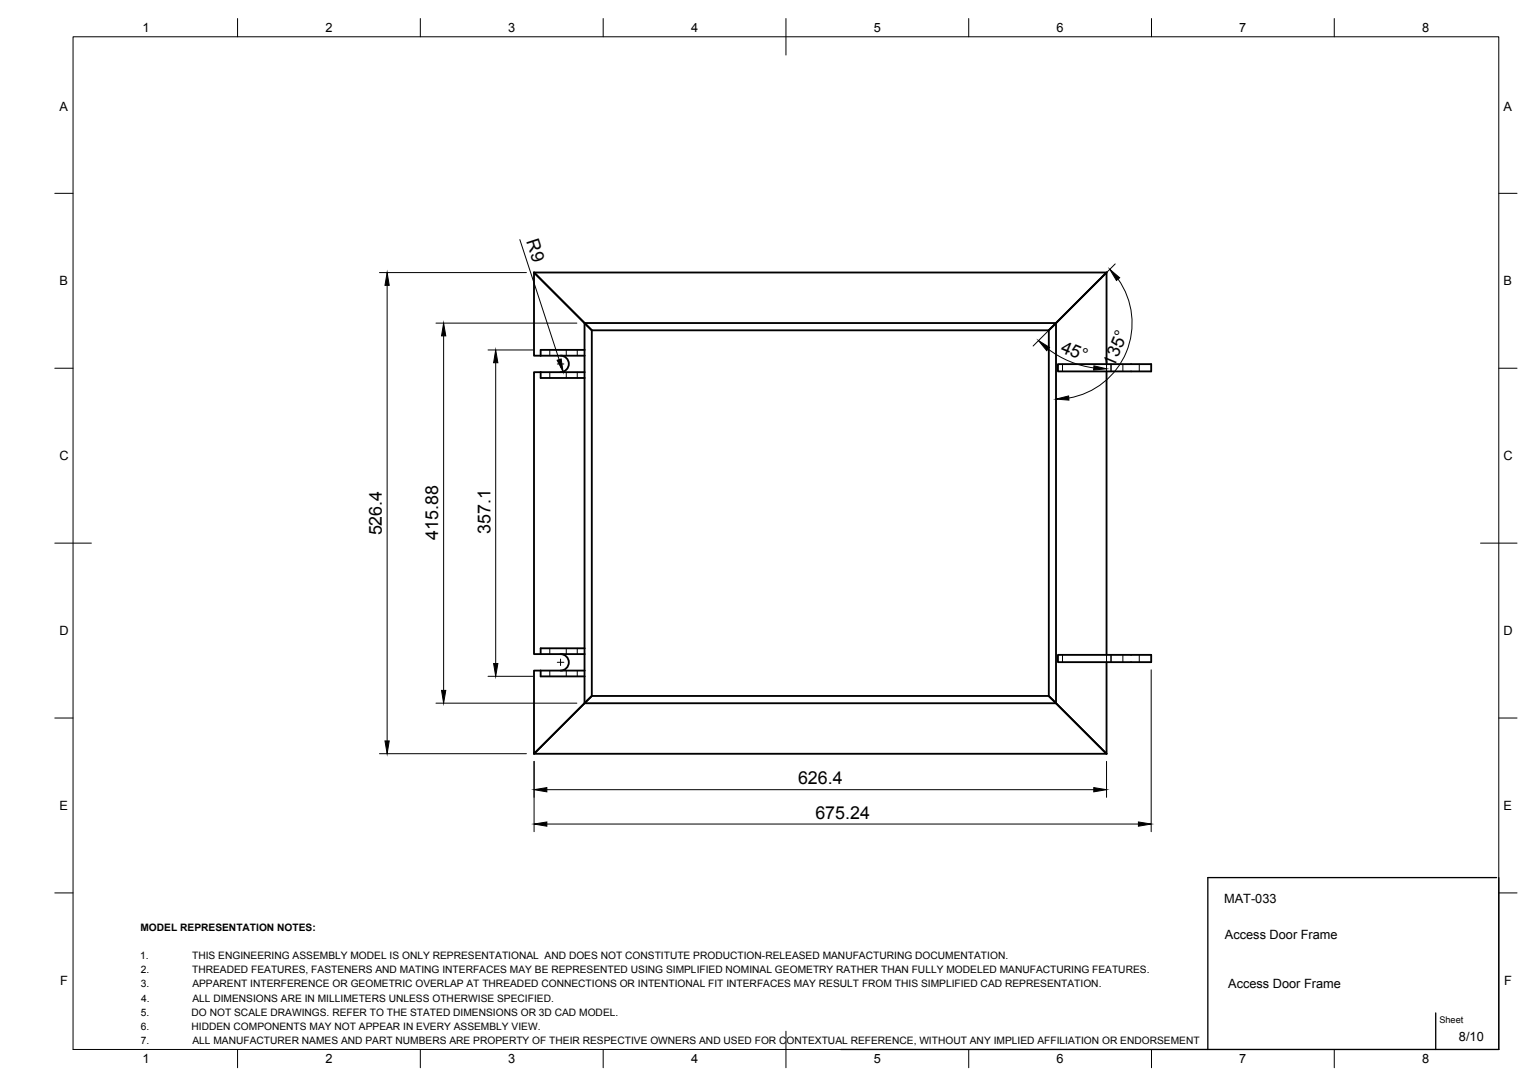
ISO-10303-21;
HEADER;
/* Generated by software containing ST-Developer
 * from STEP Tools, Inc. (www.steptools.com) 
 */

FILE_DESCRIPTION(
/* description */ ('STEP AP214'),
/* implementation_level */ '2;1');

FILE_NAME(
/* name */ 'Access Door Frame.step',
/* time_stamp */ '2026-11-14T07:13:32-08:00',
/* author */ (''),
/* organization */ (''),
/* preprocessor_version */ 'ST-DEVELOPER v20.2',
/* originating_system */ 'Autodesk Translation Framework v15.17.0.0',
/* authorisation */ '');

FILE_SCHEMA (('AUTOMOTIVE_DESIGN { 1 0 10303 214 3 1 1 }'));
ENDSEC;

DATA;
#10=MECHANICAL_DESIGN_GEOMETRIC_PRESENTATION_REPRESENTATION('',(#1305,#1306,#1307,#1308,#1309,#1310,#1311,#1312,#1313,#1314),#32903);
#644=ELLIPSE('',#16043,10.9424774388658,7.73750000000281);
#645=ELLIPSE('',#16044,11.2253201513379,7.93750000000103);
#646=ELLIPSE('',#16045,10.9424774388637,7.73750000000177);
#647=ELLIPSE('',#16047,10.9424774388587,7.73749999999781);
#648=ELLIPSE('',#16048,11.2253201513381,7.93750000000136);
#649=ELLIPSE('',#16049,10.9424774388615,7.73749999999964);
#650=ELLIPSE('',#16060,10.9424774388615,7.73749999999999);
#651=ELLIPSE('',#16061,11.2253201513371,7.93750000000052);
#652=ELLIPSE('',#16062,10.9424774388621,7.73750000000035);
#653=ELLIPSE('',#16064,10.9424774388604,7.73749999999896);
#654=ELLIPSE('',#16065,11.2253201513326,7.93749999999674);
#655=ELLIPSE('',#16066,10.9424774388621,7.73750000000041);
#656=ELLIPSE('',#16077,10.9424774388579,7.73749999999704);
#657=ELLIPSE('',#16078,11.2253201513353,7.9374999999993);
#658=ELLIPSE('',#16079,10.9424774388611,7.73749999999964);
#659=ELLIPSE('',#16081,10.9424774388619,7.73750000000076);
#660=ELLIPSE('',#16082,11.2253201513349,7.93749999999867);
#661=ELLIPSE('',#16083,10.942477438863,7.73750000000083);
#662=ELLIPSE('',#16160,10.9424774388598,7.7374999999982);
#663=ELLIPSE('',#16164,10.9424774388633,7.73750000000104);
#664=ELLIPSE('',#16165,11.225320151339,7.9375000000018);
#665=ELLIPSE('',#16166,10.9424774388576,7.73749999999669);
#666=ELLIPSE('',#16168,10.9424774388584,7.73749999999717);
#667=ELLIPSE('',#16169,11.2253201513371,7.93750000000039);
#674=SHAPE_REPRESENTATION_RELATIONSHIP('SRR','None',#33016,#688);
#688=ADVANCED_BREP_SHAPE_REPRESENTATION('',(#1394,#1395,#1396,#1397,#1398,
#1399,#1400,#1401,#1402,#1403),#32891);
#820=CIRCLE('',#16094,9.00000000000001);
#821=CIRCLE('',#16095,9.00000000000001);
#822=CIRCLE('',#16097,22.);
#823=CIRCLE('',#16098,22.);
#824=CIRCLE('',#16100,5.);
#825=CIRCLE('',#16101,5.);
#826=CIRCLE('',#16109,9.00000000000001);
#827=CIRCLE('',#16110,9.00000000000001);
#828=CIRCLE('',#16112,19.);
#829=CIRCLE('',#16114,19.);
#830=CIRCLE('',#16122,9.00000000000001);
#831=CIRCLE('',#16123,9.00000000000001);
#832=CIRCLE('',#16125,22.);
#833=CIRCLE('',#16126,22.);
#834=CIRCLE('',#16128,5.);
#835=CIRCLE('',#16129,5.);
#836=CIRCLE('',#16137,9.00000000000001);
#837=CIRCLE('',#16138,9.00000000000001);
#838=CIRCLE('',#16140,19.);
#839=CIRCLE('',#16142,19.);
#840=CIRCLE('',#16150,9.00000000000001);
#841=CIRCLE('',#16151,9.00000000000001);
#842=CIRCLE('',#16153,9.00000000000006);
#843=CIRCLE('',#16154,9.00000000000001);
#844=CIRCLE('',#16156,7.73750000000001);
#845=CIRCLE('',#16157,7.73750000000001);
#846=CIRCLE('',#16159,7.73750000000001);
#847=CIRCLE('',#16178,7.73750000000001);
#848=CIRCLE('',#16185,9.00000000000001);
#849=CIRCLE('',#16186,9.00000000000001);
#850=CIRCLE('',#16188,19.);
#851=CIRCLE('',#16190,19.);
#852=CIRCLE('',#16198,9.00000000000001);
#853=CIRCLE('',#16199,9.00000000000001);
#854=CIRCLE('',#16201,19.);
#855=CIRCLE('',#16203,19.);
#1141=CYLINDRICAL_SURFACE('',#16053,7.73749999999998);
#1142=CYLINDRICAL_SURFACE('',#16055,7.93749999999999);
#1143=CYLINDRICAL_SURFACE('',#16057,7.73750000000001);
#1144=CYLINDRICAL_SURFACE('',#16070,7.73749999999998);
#1145=CYLINDRICAL_SURFACE('',#16072,7.93750000000002);
#1146=CYLINDRICAL_SURFACE('',#16074,7.73750000000001);
#1147=CYLINDRICAL_SURFACE('',#16087,7.73749999999998);
#1148=CYLINDRICAL_SURFACE('',#16089,7.93750000000002);
#1149=CYLINDRICAL_SURFACE('',#16091,7.73750000000001);
#1150=CYLINDRICAL_SURFACE('',#16093,9.00000000000001);
#1151=CYLINDRICAL_SURFACE('',#16096,22.);
#1152=CYLINDRICAL_SURFACE('',#16099,5.);
#1153=CYLINDRICAL_SURFACE('',#16108,9.00000000000001);
#1154=CYLINDRICAL_SURFACE('',#16118,19.);
#1155=CYLINDRICAL_SURFACE('',#16121,9.00000000000001);
#1156=CYLINDRICAL_SURFACE('',#16124,22.);
#1157=CYLINDRICAL_SURFACE('',#16127,5.);
#1158=CYLINDRICAL_SURFACE('',#16136,9.00000000000001);
#1159=CYLINDRICAL_SURFACE('',#16146,19.);
#1160=CYLINDRICAL_SURFACE('',#16149,9.00000000000001);
#1161=CYLINDRICAL_SURFACE('',#16152,9.00000000000006);
#1162=CYLINDRICAL_SURFACE('',#16155,7.73750000000001);
#1163=CYLINDRICAL_SURFACE('',#16158,7.73750000000001);
#1164=CYLINDRICAL_SURFACE('',#16173,7.73749999999998);
#1165=CYLINDRICAL_SURFACE('',#16175,7.93749999999999);
#1166=CYLINDRICAL_SURFACE('',#16177,7.73750000000001);
#1167=CYLINDRICAL_SURFACE('',#16184,9.00000000000001);
#1168=CYLINDRICAL_SURFACE('',#16194,19.);
#1169=CYLINDRICAL_SURFACE('',#16197,9.00000000000001);
#1170=CYLINDRICAL_SURFACE('',#16207,19.);
#1305=STYLED_ITEM('',(#33098),#1394);
#1306=STYLED_ITEM('',(#33098),#1395);
#1307=STYLED_ITEM('',(#33098),#1396);
#1308=STYLED_ITEM('',(#33098),#1397);
#1309=STYLED_ITEM('',(#33098),#1398);
#1310=STYLED_ITEM('',(#33098),#1399);
#1311=STYLED_ITEM('',(#33098),#1400);
#1312=STYLED_ITEM('',(#33098),#1401);
#1313=STYLED_ITEM('',(#33098),#1402);
#1314=STYLED_ITEM('',(#33098),#1403);
#1394=MANIFOLD_SOLID_BREP('Body1',#15553);
#1395=MANIFOLD_SOLID_BREP('Body2',#15554);
#1396=MANIFOLD_SOLID_BREP('Body3',#15555);
#1397=MANIFOLD_SOLID_BREP('Body4',#15556);
#1398=MANIFOLD_SOLID_BREP('Body5',#15557);
#1399=MANIFOLD_SOLID_BREP('Body6',#15558);
#1400=MANIFOLD_SOLID_BREP('Body7',#15559);
#1401=MANIFOLD_SOLID_BREP('Body8',#15560);
#1402=MANIFOLD_SOLID_BREP('Body9',#15561);
#1403=MANIFOLD_SOLID_BREP('Body10',#15562);
#1579=FACE_BOUND('',#2856,.T.);
#1580=FACE_BOUND('',#2858,.T.);
#1581=FACE_BOUND('',#2861,.T.);
#1582=FACE_BOUND('',#2863,.T.);
#1583=FACE_BOUND('',#2878,.T.);
#1584=FACE_BOUND('',#2880,.T.);
#1585=FACE_BOUND('',#2883,.T.);
#1586=FACE_BOUND('',#2885,.T.);
#1587=FACE_BOUND('',#2915,.T.);
#1588=FACE_BOUND('',#2917,.T.);
#1589=FACE_BOUND('',#2926,.T.);
#1590=FACE_BOUND('',#2928,.T.);
#1810=FACE_OUTER_BOUND('',#2815,.T.);
#1811=FACE_OUTER_BOUND('',#2816,.T.);
#1812=FACE_OUTER_BOUND('',#2817,.T.);
#1813=FACE_OUTER_BOUND('',#2818,.T.);
#1814=FACE_OUTER_BOUND('',#2819,.T.);
#1815=FACE_OUTER_BOUND('',#2820,.T.);
#1816=FACE_OUTER_BOUND('',#2821,.T.);
#1817=FACE_OUTER_BOUND('',#2822,.T.);
#1818=FACE_OUTER_BOUND('',#2823,.T.);
#1819=FACE_OUTER_BOUND('',#2824,.T.);
#1820=FACE_OUTER_BOUND('',#2825,.T.);
#1821=FACE_OUTER_BOUND('',#2826,.T.);
#1822=FACE_OUTER_BOUND('',#2827,.T.);
#1823=FACE_OUTER_BOUND('',#2828,.T.);
#1824=FACE_OUTER_BOUND('',#2829,.T.);
#1825=FACE_OUTER_BOUND('',#2830,.T.);
#1826=FACE_OUTER_BOUND('',#2831,.T.);
#1827=FACE_OUTER_BOUND('',#2832,.T.);
#1828=FACE_OUTER_BOUND('',#2833,.T.);
#1829=FACE_OUTER_BOUND('',#2834,.T.);
#1830=FACE_OUTER_BOUND('',#2835,.T.);
#1831=FACE_OUTER_BOUND('',#2836,.T.);
#1832=FACE_OUTER_BOUND('',#2837,.T.);
#1833=FACE_OUTER_BOUND('',#2838,.T.);
#1834=FACE_OUTER_BOUND('',#2839,.T.);
#1835=FACE_OUTER_BOUND('',#2840,.T.);
#1836=FACE_OUTER_BOUND('',#2841,.T.);
#1837=FACE_OUTER_BOUND('',#2842,.T.);
#1838=FACE_OUTER_BOUND('',#2843,.T.);
#1839=FACE_OUTER_BOUND('',#2844,.T.);
#1840=FACE_OUTER_BOUND('',#2845,.T.);
#1841=FACE_OUTER_BOUND('',#2846,.T.);
#1842=FACE_OUTER_BOUND('',#2847,.T.);
#1843=FACE_OUTER_BOUND('',#2848,.T.);
#1844=FACE_OUTER_BOUND('',#2849,.T.);
#1845=FACE_OUTER_BOUND('',#2850,.T.);
#1846=FACE_OUTER_BOUND('',#2851,.T.);
#1847=FACE_OUTER_BOUND('',#2852,.T.);
#1848=FACE_OUTER_BOUND('',#2853,.T.);
#1849=FACE_OUTER_BOUND('',#2854,.T.);
#1850=FACE_OUTER_BOUND('',#2855,.T.);
#1851=FACE_OUTER_BOUND('',#2857,.T.);
#1852=FACE_OUTER_BOUND('',#2859,.T.);
#1853=FACE_OUTER_BOUND('',#2860,.T.);
#1854=FACE_OUTER_BOUND('',#2862,.T.);
#1855=FACE_OUTER_BOUND('',#2864,.T.);
#1856=FACE_OUTER_BOUND('',#2865,.T.);
#1857=FACE_OUTER_BOUND('',#2866,.T.);
#1858=FACE_OUTER_BOUND('',#2867,.T.);
#1859=FACE_OUTER_BOUND('',#2868,.T.);
#1860=FACE_OUTER_BOUND('',#2869,.T.);
#1861=FACE_OUTER_BOUND('',#2870,.T.);
#1862=FACE_OUTER_BOUND('',#2871,.T.);
#1863=FACE_OUTER_BOUND('',#2872,.T.);
#1864=FACE_OUTER_BOUND('',#2873,.T.);
#1865=FACE_OUTER_BOUND('',#2874,.T.);
#1866=FACE_OUTER_BOUND('',#2875,.T.);
#1867=FACE_OUTER_BOUND('',#2876,.T.);
#1868=FACE_OUTER_BOUND('',#2877,.T.);
#1869=FACE_OUTER_BOUND('',#2879,.T.);
#1870=FACE_OUTER_BOUND('',#2881,.T.);
#1871=FACE_OUTER_BOUND('',#2882,.T.);
#1872=FACE_OUTER_BOUND('',#2884,.T.);
#1873=FACE_OUTER_BOUND('',#2886,.T.);
#1874=FACE_OUTER_BOUND('',#2887,.T.);
#1875=FACE_OUTER_BOUND('',#2888,.T.);
#1876=FACE_OUTER_BOUND('',#2889,.T.);
#1877=FACE_OUTER_BOUND('',#2890,.T.);
#1878=FACE_OUTER_BOUND('',#2891,.T.);
#1879=FACE_OUTER_BOUND('',#2892,.T.);
#1880=FACE_OUTER_BOUND('',#2893,.T.);
#1881=FACE_OUTER_BOUND('',#2894,.T.);
#1882=FACE_OUTER_BOUND('',#2895,.T.);
#1883=FACE_OUTER_BOUND('',#2896,.T.);
#1884=FACE_OUTER_BOUND('',#2897,.T.);
#1885=FACE_OUTER_BOUND('',#2898,.T.);
#1886=FACE_OUTER_BOUND('',#2899,.T.);
#1887=FACE_OUTER_BOUND('',#2900,.T.);
#1888=FACE_OUTER_BOUND('',#2901,.T.);
#1889=FACE_OUTER_BOUND('',#2902,.T.);
#1890=FACE_OUTER_BOUND('',#2903,.T.);
#1891=FACE_OUTER_BOUND('',#2904,.T.);
#1892=FACE_OUTER_BOUND('',#2905,.T.);
#1893=FACE_OUTER_BOUND('',#2906,.T.);
#1894=FACE_OUTER_BOUND('',#2907,.T.);
#1895=FACE_OUTER_BOUND('',#2908,.T.);
#1896=FACE_OUTER_BOUND('',#2909,.T.);
#1897=FACE_OUTER_BOUND('',#2910,.T.);
#1898=FACE_OUTER_BOUND('',#2911,.T.);
#1899=FACE_OUTER_BOUND('',#2912,.T.);
#1900=FACE_OUTER_BOUND('',#2913,.T.);
#1901=FACE_OUTER_BOUND('',#2914,.T.);
#1902=FACE_OUTER_BOUND('',#2916,.T.);
#1903=FACE_OUTER_BOUND('',#2918,.T.);
#1904=FACE_OUTER_BOUND('',#2919,.T.);
#1905=FACE_OUTER_BOUND('',#2920,.T.);
#1906=FACE_OUTER_BOUND('',#2921,.T.);
#1907=FACE_OUTER_BOUND('',#2922,.T.);
#1908=FACE_OUTER_BOUND('',#2923,.T.);
#1909=FACE_OUTER_BOUND('',#2924,.T.);
#1910=FACE_OUTER_BOUND('',#2925,.T.);
#1911=FACE_OUTER_BOUND('',#2927,.T.);
#1912=FACE_OUTER_BOUND('',#2929,.T.);
#1913=FACE_OUTER_BOUND('',#2930,.T.);
#1914=FACE_OUTER_BOUND('',#2931,.T.);
#1915=FACE_OUTER_BOUND('',#2932,.T.);
#1916=FACE_OUTER_BOUND('',#2933,.T.);
#1917=FACE_OUTER_BOUND('',#2934,.T.);
#2815=EDGE_LOOP('',(#10543,#10544,#10545,#10546,#10547,#10548,#10549,#10550,
#10551));
#2816=EDGE_LOOP('',(#10552,#10553,#10554,#10555,#10556,#10557,#10558,#10559,
#10560));
#2817=EDGE_LOOP('',(#10561,#10562,#10563,#10564));
#2818=EDGE_LOOP('',(#10565,#10566,#10567,#10568));
#2819=EDGE_LOOP('',(#10569,#10570,#10571,#10572));
#2820=EDGE_LOOP('',(#10573,#10574,#10575,#10576));
#2821=EDGE_LOOP('',(#10577,#10578,#10579,#10580));
#2822=EDGE_LOOP('',(#10581,#10582,#10583,#10584));
#2823=EDGE_LOOP('',(#10585,#10586,#10587,#10588));
#2824=EDGE_LOOP('',(#10589,#10590,#10591,#10592));
#2825=EDGE_LOOP('',(#10593,#10594,#10595,#10596));
#2826=EDGE_LOOP('',(#10597,#10598,#10599,#10600,#10601,#10602,#10603,#10604,
#10605));
#2827=EDGE_LOOP('',(#10606,#10607,#10608,#10609,#10610,#10611,#10612,#10613,
#10614));
#2828=EDGE_LOOP('',(#10615,#10616,#10617,#10618));
#2829=EDGE_LOOP('',(#10619,#10620,#10621,#10622));
#2830=EDGE_LOOP('',(#10623,#10624,#10625,#10626));
#2831=EDGE_LOOP('',(#10627,#10628,#10629,#10630));
#2832=EDGE_LOOP('',(#10631,#10632,#10633,#10634));
#2833=EDGE_LOOP('',(#10635,#10636,#10637,#10638));
#2834=EDGE_LOOP('',(#10639,#10640,#10641,#10642));
#2835=EDGE_LOOP('',(#10643,#10644,#10645,#10646));
#2836=EDGE_LOOP('',(#10647,#10648,#10649,#10650));
#2837=EDGE_LOOP('',(#10651,#10652,#10653,#10654,#10655,#10656,#10657,#10658,
#10659));
#2838=EDGE_LOOP('',(#10660,#10661,#10662,#10663,#10664,#10665,#10666,#10667,
#10668));
#2839=EDGE_LOOP('',(#10669,#10670,#10671,#10672));
#2840=EDGE_LOOP('',(#10673,#10674,#10675,#10676));
#2841=EDGE_LOOP('',(#10677,#10678,#10679,#10680));
#2842=EDGE_LOOP('',(#10681,#10682,#10683,#10684));
#2843=EDGE_LOOP('',(#10685,#10686,#10687,#10688));
#2844=EDGE_LOOP('',(#10689,#10690,#10691,#10692));
#2845=EDGE_LOOP('',(#10693,#10694,#10695,#10696));
#2846=EDGE_LOOP('',(#10697,#10698,#10699,#10700));
#2847=EDGE_LOOP('',(#10701,#10702,#10703,#10704));
#2848=EDGE_LOOP('',(#10705,#10706,#10707,#10708));
#2849=EDGE_LOOP('',(#10709,#10710,#10711,#10712));
#2850=EDGE_LOOP('',(#10713,#10714,#10715,#10716));
#2851=EDGE_LOOP('',(#10717,#10718,#10719,#10720));
#2852=EDGE_LOOP('',(#10721,#10722,#10723,#10724));
#2853=EDGE_LOOP('',(#10725,#10726,#10727,#10728));
#2854=EDGE_LOOP('',(#10729,#10730,#10731,#10732));
#2855=EDGE_LOOP('',(#10733,#10734,#10735,#10736,#10737,#10738));
#2856=EDGE_LOOP('',(#10739));
#2857=EDGE_LOOP('',(#10740,#10741,#10742,#10743,#10744,#10745));
#2858=EDGE_LOOP('',(#10746));
#2859=EDGE_LOOP('',(#10747,#10748,#10749,#10750));
#2860=EDGE_LOOP('',(#10751,#10752,#10753,#10754,#10755,#10756));
#2861=EDGE_LOOP('',(#10757));
#2862=EDGE_LOOP('',(#10758,#10759,#10760,#10761,#10762,#10763));
#2863=EDGE_LOOP('',(#10764));
#2864=EDGE_LOOP('',(#10765,#10766,#10767,#10768));
#2865=EDGE_LOOP('',(#10769,#10770,#10771,#10772));
#2866=EDGE_LOOP('',(#10773,#10774,#10775,#10776));
#2867=EDGE_LOOP('',(#10777,#10778,#10779,#10780));
#2868=EDGE_LOOP('',(#10781,#10782,#10783,#10784));
#2869=EDGE_LOOP('',(#10785,#10786,#10787,#10788));
#2870=EDGE_LOOP('',(#10789,#10790,#10791,#10792));
#2871=EDGE_LOOP('',(#10793,#10794,#10795,#10796));
#2872=EDGE_LOOP('',(#10797,#10798,#10799,#10800));
#2873=EDGE_LOOP('',(#10801,#10802,#10803,#10804));
#2874=EDGE_LOOP('',(#10805,#10806,#10807,#10808));
#2875=EDGE_LOOP('',(#10809,#10810,#10811,#10812));
#2876=EDGE_LOOP('',(#10813,#10814,#10815,#10816));
#2877=EDGE_LOOP('',(#10817,#10818,#10819,#10820,#10821,#10822));
#2878=EDGE_LOOP('',(#10823));
#2879=EDGE_LOOP('',(#10824,#10825,#10826,#10827,#10828,#10829));
#2880=EDGE_LOOP('',(#10830));
#2881=EDGE_LOOP('',(#10831,#10832,#10833,#10834));
#2882=EDGE_LOOP('',(#10835,#10836,#10837,#10838,#10839,#10840));
#2883=EDGE_LOOP('',(#10841));
#2884=EDGE_LOOP('',(#10842,#10843,#10844,#10845,#10846,#10847));
#2885=EDGE_LOOP('',(#10848));
#2886=EDGE_LOOP('',(#10849,#10850,#10851,#10852));
#2887=EDGE_LOOP('',(#10853,#10854,#10855,#10856));
#2888=EDGE_LOOP('',(#10857,#10858,#10859,#10860));
#2889=EDGE_LOOP('',(#10861,#10862,#10863,#10864));
#2890=EDGE_LOOP('',(#10865,#10866,#10867,#10868));
#2891=EDGE_LOOP('',(#10869,#10870,#10871,#10872));
#2892=EDGE_LOOP('',(#10873,#10874,#10875,#10876));
#2893=EDGE_LOOP('',(#10877,#10878,#10879,#10880));
#2894=EDGE_LOOP('',(#10881,#10882,#10883,#10884));
#2895=EDGE_LOOP('',(#10885,#10886,#10887,#10888));
#2896=EDGE_LOOP('',(#10889,#10890,#10891,#10892));
#2897=EDGE_LOOP('',(#10893,#10894,#10895,#10896));
#2898=EDGE_LOOP('',(#10897,#10898,#10899,#10900,#10901,#10902,#10903,#10904,
#10905));
#2899=EDGE_LOOP('',(#10906,#10907,#10908,#10909,#10910,#10911,#10912,#10913,
#10914));
#2900=EDGE_LOOP('',(#10915,#10916,#10917,#10918,#10919,#10920,#10921,#10922,
#10923,#10924,#10925,#10926));
#2901=EDGE_LOOP('',(#10927,#10928,#10929,#10930));
#2902=EDGE_LOOP('',(#10931,#10932,#10933,#10934));
#2903=EDGE_LOOP('',(#10935,#10936,#10937,#10938));
#2904=EDGE_LOOP('',(#10939,#10940,#10941,#10942));
#2905=EDGE_LOOP('',(#10943,#10944,#10945,#10946));
#2906=EDGE_LOOP('',(#10947,#10948,#10949,#10950,#10951,#10952,#10953,#10954,
#10955,#10956,#10957,#10958));
#2907=EDGE_LOOP('',(#10959,#10960,#10961,#10962));
#2908=EDGE_LOOP('',(#10963,#10964,#10965,#10966));
#2909=EDGE_LOOP('',(#10967,#10968,#10969,#10970,#10971));
#2910=EDGE_LOOP('',(#10972,#10973,#10974,#10975,#10976));
#2911=EDGE_LOOP('',(#10977,#10978,#10979,#10980,#10981));
#2912=EDGE_LOOP('',(#10982,#10983,#10984,#10985,#10986));
#2913=EDGE_LOOP('',(#10987,#10988,#10989,#10990));
#2914=EDGE_LOOP('',(#10991,#10992,#10993,#10994,#10995,#10996));
#2915=EDGE_LOOP('',(#10997));
#2916=EDGE_LOOP('',(#10998,#10999,#11000,#11001,#11002,#11003));
#2917=EDGE_LOOP('',(#11004));
#2918=EDGE_LOOP('',(#11005,#11006,#11007,#11008));
#2919=EDGE_LOOP('',(#11009,#11010,#11011,#11012));
#2920=EDGE_LOOP('',(#11013,#11014,#11015,#11016));
#2921=EDGE_LOOP('',(#11017,#11018,#11019,#11020));
#2922=EDGE_LOOP('',(#11021,#11022,#11023,#11024));
#2923=EDGE_LOOP('',(#11025,#11026,#11027,#11028));
#2924=EDGE_LOOP('',(#11029,#11030,#11031,#11032));
#2925=EDGE_LOOP('',(#11033,#11034,#11035,#11036,#11037,#11038));
#2926=EDGE_LOOP('',(#11039));
#2927=EDGE_LOOP('',(#11040,#11041,#11042,#11043,#11044,#11045));
#2928=EDGE_LOOP('',(#11046));
#2929=EDGE_LOOP('',(#11047,#11048,#11049,#11050));
#2930=EDGE_LOOP('',(#11051,#11052,#11053,#11054));
#2931=EDGE_LOOP('',(#11055,#11056,#11057,#11058));
#2932=EDGE_LOOP('',(#11059,#11060,#11061,#11062));
#2933=EDGE_LOOP('',(#11063,#11064,#11065,#11066));
#2934=EDGE_LOOP('',(#11067,#11068,#11069,#11070));
#3871=LINE('',#21981,#5275);
#3872=LINE('',#21983,#5276);
#3873=LINE('',#21985,#5277);
#3874=LINE('',#21987,#5278);
#3875=LINE('',#21991,#5279);
#3876=LINE('',#21995,#5280);
#3877=LINE('',#22000,#5281);
#3878=LINE('',#22002,#5282);
#3879=LINE('',#22006,#5283);
#3880=LINE('',#22010,#5284);
#3881=LINE('',#22014,#5285);
#3882=LINE('',#22015,#5286);
#3883=LINE('',#22017,#5287);
#3884=LINE('',#22018,#5288);
#3885=LINE('',#22020,#5289);
#3886=LINE('',#22022,#5290);
#3887=LINE('',#22024,#5291);
#3888=LINE('',#22026,#5292);
#3889=LINE('',#22028,#5293);
#3890=LINE('',#22030,#5294);
#3891=LINE('',#22032,#5295);
#3892=LINE('',#22037,#5296);
#3893=LINE('',#22041,#5297);
#3894=LINE('',#22045,#5298);
#3895=LINE('',#22049,#5299);
#3896=LINE('',#22051,#5300);
#3897=LINE('',#22052,#5301);
#3898=LINE('',#22056,#5302);
#3899=LINE('',#22058,#5303);
#3900=LINE('',#22060,#5304);
#3901=LINE('',#22064,#5305);
#3902=LINE('',#22068,#5306);
#3903=LINE('',#22071,#5307);
#3904=LINE('',#22073,#5308);
#3905=LINE('',#22074,#5309);
#3906=LINE('',#22076,#5310);
#3907=LINE('',#22078,#5311);
#3908=LINE('',#22080,#5312);
#3909=LINE('',#22082,#5313);
#3910=LINE('',#22084,#5314);
#3911=LINE('',#22086,#5315);
#3912=LINE('',#22088,#5316);
#3913=LINE('',#22093,#5317);
#3914=LINE('',#22097,#5318);
#3915=LINE('',#22101,#5319);
#3916=LINE('',#22105,#5320);
#3917=LINE('',#22107,#5321);
#3918=LINE('',#22108,#5322);
#3919=LINE('',#22112,#5323);
#3920=LINE('',#22114,#5324);
#3921=LINE('',#22116,#5325);
#3922=LINE('',#22120,#5326);
#3923=LINE('',#22124,#5327);
#3924=LINE('',#22127,#5328);
#3925=LINE('',#22129,#5329);
#3926=LINE('',#22130,#5330);
#3927=LINE('',#22132,#5331);
#3928=LINE('',#22134,#5332);
#3929=LINE('',#22136,#5333);
#3930=LINE('',#22138,#5334);
#3931=LINE('',#22140,#5335);
#3932=LINE('',#22142,#5336);
#3933=LINE('',#22144,#5337);
#3934=LINE('',#22150,#5338);
#3935=LINE('',#22157,#5339);
#3936=LINE('',#22160,#5340);
#3937=LINE('',#22165,#5341);
#3938=LINE('',#22169,#5342);
#3939=LINE('',#22171,#5343);
#3940=LINE('',#22172,#5344);
#3941=LINE('',#22175,#5345);
#3942=LINE('',#22177,#5346);
#3943=LINE('',#22178,#5347);
#3944=LINE('',#22181,#5348);
#3945=LINE('',#22183,#5349);
#3946=LINE('',#22184,#5350);
#3947=LINE('',#22186,#5351);
#3948=LINE('',#22187,#5352);
#3949=LINE('',#22194,#5353);
#3950=LINE('',#22199,#5354);
#3951=LINE('',#22201,#5355);
#3952=LINE('',#22203,#5356);
#3953=LINE('',#22207,#5357);
#3954=LINE('',#22208,#5358);
#3955=LINE('',#22212,#5359);
#3956=LINE('',#22214,#5360);
#3957=LINE('',#22216,#5361);
#3958=LINE('',#22220,#5362);
#3959=LINE('',#22221,#5363);
#3960=LINE('',#22223,#5364);
#3961=LINE('',#22224,#5365);
#3962=LINE('',#22226,#5366);
#3963=LINE('',#22228,#5367);
#3964=LINE('',#22230,#5368);
#3965=LINE('',#22232,#5369);
#3966=LINE('',#22238,#5370);
#3967=LINE('',#22245,#5371);
#3968=LINE('',#22248,#5372);
#3969=LINE('',#22254,#5373);
#3970=LINE('',#22257,#5374);
#3971=LINE('',#22259,#5375);
#3972=LINE('',#22260,#5376);
#3973=LINE('',#22263,#5377);
#3974=LINE('',#22265,#5378);
#3975=LINE('',#22266,#5379);
#3976=LINE('',#22269,#5380);
#3977=LINE('',#22271,#5381);
#3978=LINE('',#22272,#5382);
#3979=LINE('',#22274,#5383);
#3980=LINE('',#22275,#5384);
#3981=LINE('',#22282,#5385);
#3982=LINE('',#22287,#5386);
#3983=LINE('',#22289,#5387);
#3984=LINE('',#22291,#5388);
#3985=LINE('',#22295,#5389);
#3986=LINE('',#22296,#5390);
#3987=LINE('',#22300,#5391);
#3988=LINE('',#22302,#5392);
#3989=LINE('',#22304,#5393);
#3990=LINE('',#22308,#5394);
#3991=LINE('',#22309,#5395);
#3992=LINE('',#22311,#5396);
#3993=LINE('',#22312,#5397);
#3994=LINE('',#22314,#5398);
#3995=LINE('',#22316,#5399);
#3996=LINE('',#22318,#5400);
#3997=LINE('',#22320,#5401);
#3998=LINE('',#22327,#5402);
#3999=LINE('',#22330,#5403);
#4000=LINE('',#22336,#5404);
#4001=LINE('',#22339,#5405);
#4002=LINE('',#22345,#5406);
#4003=LINE('',#22348,#5407);
#4004=LINE('',#22354,#5408);
#4005=LINE('',#22357,#5409);
#4006=LINE('',#22360,#5410);
#4007=LINE('',#22362,#5411);
#4008=LINE('',#22363,#5412);
#4009=LINE('',#22366,#5413);
#4010=LINE('',#22368,#5414);
#4011=LINE('',#22369,#5415);
#4012=LINE('',#22373,#5416);
#4013=LINE('',#22377,#5417);
#4014=LINE('',#22381,#5418);
#4015=LINE('',#22385,#5419);
#4016=LINE('',#22387,#5420);
#4017=LINE('',#22388,#5421);
#4018=LINE('',#22391,#5422);
#4019=LINE('',#22393,#5423);
#4020=LINE('',#22395,#5424);
#4021=LINE('',#22399,#5425);
#4022=LINE('',#22402,#5426);
#4023=LINE('',#22404,#5427);
#4024=LINE('',#22406,#5428);
#4025=LINE('',#22407,#5429);
#4026=LINE('',#22408,#5430);
#4027=LINE('',#22409,#5431);
#4028=LINE('',#22410,#5432);
#4029=LINE('',#22412,#5433);
#4030=LINE('',#22414,#5434);
#4031=LINE('',#22416,#5435);
#4032=LINE('',#22418,#5436);
#4033=LINE('',#22420,#5437);
#4034=LINE('',#22422,#5438);
#4035=LINE('',#22423,#5439);
#4036=LINE('',#22424,#5440);
#4037=LINE('',#22426,#5441);
#4038=LINE('',#22427,#5442);
#4039=LINE('',#22431,#5443);
#4040=LINE('',#22433,#5444);
#4041=LINE('',#22442,#5445);
#4042=LINE('',#22447,#5446);
#4043=LINE('',#22449,#5447);
#4044=LINE('',#22451,#5448);
#4045=LINE('',#22455,#5449);
#4046=LINE('',#22456,#5450);
#4047=LINE('',#22460,#5451);
#4048=LINE('',#22462,#5452);
#4049=LINE('',#22464,#5453);
#4050=LINE('',#22468,#5454);
#4051=LINE('',#22469,#5455);
#4052=LINE('',#22471,#5456);
#4053=LINE('',#22472,#5457);
#4054=LINE('',#22474,#5458);
#4055=LINE('',#22476,#5459);
#4056=LINE('',#22478,#5460);
#4057=LINE('',#22480,#5461);
#4058=LINE('',#22486,#5462);
#4059=LINE('',#22491,#5463);
#4060=LINE('',#22493,#5464);
#4061=LINE('',#22495,#5465);
#4062=LINE('',#22499,#5466);
#4063=LINE('',#22500,#5467);
#4064=LINE('',#22504,#5468);
#4065=LINE('',#22506,#5469);
#4066=LINE('',#22508,#5470);
#4067=LINE('',#22512,#5471);
#4068=LINE('',#22513,#5472);
#4069=LINE('',#22515,#5473);
#4070=LINE('',#22516,#5474);
#4071=LINE('',#22518,#5475);
#4072=LINE('',#22520,#5476);
#4073=LINE('',#22522,#5477);
#4074=LINE('',#22524,#5478);
#5275=VECTOR('',#17875,1000.);
#5276=VECTOR('',#17876,1000.);
#5277=VECTOR('',#17877,1000.);
#5278=VECTOR('',#17878,1000.);
#5279=VECTOR('',#17881,1000.);
#5280=VECTOR('',#17884,1000.);
#5281=VECTOR('',#17889,1000.);
#5282=VECTOR('',#17890,1000.);
#5283=VECTOR('',#17893,1000.);
#5284=VECTOR('',#17896,1000.);
#5285=VECTOR('',#17899,1000.);
#5286=VECTOR('',#17900,1000.);
#5287=VECTOR('',#17903,1000.);
#5288=VECTOR('',#17904,1000.);
#5289=VECTOR('',#17907,1000.);
#5290=VECTOR('',#17910,1000.);
#5291=VECTOR('',#17913,1000.);
#5292=VECTOR('',#17916,1000.);
#5293=VECTOR('',#17919,1000.);
#5294=VECTOR('',#17922,1000.);
#5295=VECTOR('',#17925,1000.);
#5296=VECTOR('',#17930,1000.);
#5297=VECTOR('',#17933,1000.);
#5298=VECTOR('',#17936,1000.);
#5299=VECTOR('',#17939,1000.);
#5300=VECTOR('',#17940,1000.);
#5301=VECTOR('',#17941,1000.);
#5302=VECTOR('',#17944,1000.);
#5303=VECTOR('',#17945,1000.);
#5304=VECTOR('',#17946,1000.);
#5305=VECTOR('',#17949,1000.);
#5306=VECTOR('',#17952,1000.);
#5307=VECTOR('',#17955,1000.);
#5308=VECTOR('',#17958,1000.);
#5309=VECTOR('',#17959,1000.);
#5310=VECTOR('',#17962,1000.);
#5311=VECTOR('',#17965,1000.);
#5312=VECTOR('',#17968,1000.);
#5313=VECTOR('',#17971,1000.);
#5314=VECTOR('',#17974,1000.);
#5315=VECTOR('',#17977,1000.);
#5316=VECTOR('',#17980,1000.);
#5317=VECTOR('',#17985,1000.);
#5318=VECTOR('',#17988,1000.);
#5319=VECTOR('',#17991,1000.);
#5320=VECTOR('',#17994,1000.);
#5321=VECTOR('',#17995,1000.);
#5322=VECTOR('',#17996,1000.);
#5323=VECTOR('',#17999,1000.);
#5324=VECTOR('',#18000,1000.);
#5325=VECTOR('',#18001,1000.);
#5326=VECTOR('',#18004,1000.);
#5327=VECTOR('',#18007,1000.);
#5328=VECTOR('',#18010,1000.);
#5329=VECTOR('',#18013,1000.);
#5330=VECTOR('',#18014,1000.);
#5331=VECTOR('',#18017,1000.);
#5332=VECTOR('',#18020,1000.);
#5333=VECTOR('',#18023,1000.);
#5334=VECTOR('',#18026,1000.);
#5335=VECTOR('',#18029,1000.);
#5336=VECTOR('',#18032,1000.);
#5337=VECTOR('',#18035,1000.);
#5338=VECTOR('',#18042,9.00000000000001);
#5339=VECTOR('',#18049,1000.);
#5340=VECTOR('',#18052,1000.);
#5341=VECTOR('',#18057,1000.);
#5342=VECTOR('',#18062,1000.);
#5343=VECTOR('',#18063,1000.);
#5344=VECTOR('',#18064,1000.);
#5345=VECTOR('',#18067,1000.);
#5346=VECTOR('',#18068,1000.);
#5347=VECTOR('',#18069,1000.);
#5348=VECTOR('',#18072,1000.);
#5349=VECTOR('',#18073,1000.);
#5350=VECTOR('',#18074,1000.);
#5351=VECTOR('',#18077,1000.);
#5352=VECTOR('',#18078,1000.);
#5353=VECTOR('',#18087,9.00000000000001);
#5354=VECTOR('',#18092,1000.);
#5355=VECTOR('',#18093,1000.);
#5356=VECTOR('',#18094,1000.);
#5357=VECTOR('',#18097,1000.);
#5358=VECTOR('',#18098,1000.);
#5359=VECTOR('',#18101,1000.);
#5360=VECTOR('',#18102,1000.);
#5361=VECTOR('',#18103,1000.);
#5362=VECTOR('',#18106,1000.);
#5363=VECTOR('',#18107,1000.);
#5364=VECTOR('',#18110,1000.);
#5365=VECTOR('',#18111,1000.);
#5366=VECTOR('',#18114,1000.);
#5367=VECTOR('',#18117,1000.);
#5368=VECTOR('',#18120,1000.);
#5369=VECTOR('',#18123,1000.);
#5370=VECTOR('',#18130,9.00000000000001);
#5371=VECTOR('',#18137,1000.);
#5372=VECTOR('',#18140,1000.);
#5373=VECTOR('',#18147,1000.);
#5374=VECTOR('',#18150,1000.);
#5375=VECTOR('',#18151,1000.);
#5376=VECTOR('',#18152,1000.);
#5377=VECTOR('',#18155,1000.);
#5378=VECTOR('',#18156,1000.);
#5379=VECTOR('',#18157,1000.);
#5380=VECTOR('',#18160,1000.);
#5381=VECTOR('',#18161,1000.);
#5382=VECTOR('',#18162,1000.);
#5383=VECTOR('',#18165,1000.);
#5384=VECTOR('',#18166,1000.);
#5385=VECTOR('',#18175,9.00000000000001);
#5386=VECTOR('',#18180,1000.);
#5387=VECTOR('',#18181,1000.);
#5388=VECTOR('',#18182,1000.);
#5389=VECTOR('',#18185,1000.);
#5390=VECTOR('',#18186,1000.);
#5391=VECTOR('',#18189,1000.);
#5392=VECTOR('',#18190,1000.);
#5393=VECTOR('',#18191,1000.);
#5394=VECTOR('',#18194,1000.);
#5395=VECTOR('',#18195,1000.);
#5396=VECTOR('',#18198,1000.);
#5397=VECTOR('',#18199,1000.);
#5398=VECTOR('',#18202,1000.);
#5399=VECTOR('',#18205,1000.);
#5400=VECTOR('',#18208,1000.);
#5401=VECTOR('',#18211,1000.);
#5402=VECTOR('',#18218,1000.);
#5403=VECTOR('',#18221,1000.);
#5404=VECTOR('',#18226,1000.);
#5405=VECTOR('',#18229,1000.);
#5406=VECTOR('',#18234,1000.);
#5407=VECTOR('',#18237,1000.);
#5408=VECTOR('',#18242,1000.);
#5409=VECTOR('',#18245,1000.);
#5410=VECTOR('',#18248,1000.);
#5411=VECTOR('',#18249,1000.);
#5412=VECTOR('',#18250,1000.);
#5413=VECTOR('',#18253,1000.);
#5414=VECTOR('',#18254,1000.);
#5415=VECTOR('',#18255,1000.);
#5416=VECTOR('',#18258,1000.);
#5417=VECTOR('',#18261,1000.);
#5418=VECTOR('',#18264,1000.);
#5419=VECTOR('',#18267,1000.);
#5420=VECTOR('',#18268,1000.);
#5421=VECTOR('',#18269,1000.);
#5422=VECTOR('',#18272,1000.);
#5423=VECTOR('',#18273,1000.);
#5424=VECTOR('',#18274,1000.);
#5425=VECTOR('',#18277,1000.);
#5426=VECTOR('',#18280,1000.);
#5427=VECTOR('',#18283,1000.);
#5428=VECTOR('',#18284,1000.);
#5429=VECTOR('',#18285,1000.);
#5430=VECTOR('',#18286,1000.);
#5431=VECTOR('',#18287,1000.);
#5432=VECTOR('',#18288,1000.);
#5433=VECTOR('',#18291,1000.);
#5434=VECTOR('',#18294,1000.);
#5435=VECTOR('',#18297,1000.);
#5436=VECTOR('',#18300,1000.);
#5437=VECTOR('',#18303,1000.);
#5438=VECTOR('',#18306,1000.);
#5439=VECTOR('',#18307,1000.);
#5440=VECTOR('',#18308,1000.);
#5441=VECTOR('',#18309,1000.);
#5442=VECTOR('',#18310,1000.);
#5443=VECTOR('',#18315,1000.);
#5444=VECTOR('',#18318,1000.);
#5445=VECTOR('',#18331,9.00000000000001);
#5446=VECTOR('',#18336,1000.);
#5447=VECTOR('',#18337,1000.);
#5448=VECTOR('',#18338,1000.);
#5449=VECTOR('',#18341,1000.);
#5450=VECTOR('',#18342,1000.);
#5451=VECTOR('',#18345,1000.);
#5452=VECTOR('',#18346,1000.);
#5453=VECTOR('',#18347,1000.);
#5454=VECTOR('',#18350,1000.);
#5455=VECTOR('',#18351,1000.);
#5456=VECTOR('',#18354,1000.);
#5457=VECTOR('',#18355,1000.);
#5458=VECTOR('',#18358,1000.);
#5459=VECTOR('',#18361,1000.);
#5460=VECTOR('',#18364,1000.);
#5461=VECTOR('',#18367,1000.);
#5462=VECTOR('',#18374,9.00000000000001);
#5463=VECTOR('',#18379,1000.);
#5464=VECTOR('',#18380,1000.);
#5465=VECTOR('',#18381,1000.);
#5466=VECTOR('',#18384,1000.);
#5467=VECTOR('',#18385,1000.);
#5468=VECTOR('',#18388,1000.);
#5469=VECTOR('',#18389,1000.);
#5470=VECTOR('',#18390,1000.);
#5471=VECTOR('',#18393,1000.);
#5472=VECTOR('',#18394,1000.);
#5473=VECTOR('',#18397,1000.);
#5474=VECTOR('',#18398,1000.);
#5475=VECTOR('',#18401,1000.);
#5476=VECTOR('',#18404,1000.);
#5477=VECTOR('',#18407,1000.);
#5478=VECTOR('',#18410,1000.);
#6693=VERTEX_POINT('',#21979);
#6694=VERTEX_POINT('',#21980);
#6695=VERTEX_POINT('',#21982);
#6696=VERTEX_POINT('',#21984);
#6697=VERTEX_POINT('',#21986);
#6698=VERTEX_POINT('',#21988);
#6699=VERTEX_POINT('',#21990);
#6700=VERTEX_POINT('',#21992);
#6701=VERTEX_POINT('',#21994);
#6702=VERTEX_POINT('',#21998);
#6703=VERTEX_POINT('',#21999);
#6704=VERTEX_POINT('',#22001);
#6705=VERTEX_POINT('',#22003);
#6706=VERTEX_POINT('',#22005);
#6707=VERTEX_POINT('',#22007);
#6708=VERTEX_POINT('',#22009);
#6709=VERTEX_POINT('',#22011);
#6710=VERTEX_POINT('',#22013);
#6711=VERTEX_POINT('',#22035);
#6712=VERTEX_POINT('',#22036);
#6713=VERTEX_POINT('',#22038);
#6714=VERTEX_POINT('',#22040);
#6715=VERTEX_POINT('',#22042);
#6716=VERTEX_POINT('',#22044);
#6717=VERTEX_POINT('',#22046);
#6718=VERTEX_POINT('',#22048);
#6719=VERTEX_POINT('',#22050);
#6720=VERTEX_POINT('',#22054);
#6721=VERTEX_POINT('',#22055);
#6722=VERTEX_POINT('',#22057);
#6723=VERTEX_POINT('',#22059);
#6724=VERTEX_POINT('',#22061);
#6725=VERTEX_POINT('',#22063);
#6726=VERTEX_POINT('',#22065);
#6727=VERTEX_POINT('',#22067);
#6728=VERTEX_POINT('',#22069);
#6729=VERTEX_POINT('',#22091);
#6730=VERTEX_POINT('',#22092);
#6731=VERTEX_POINT('',#22094);
#6732=VERTEX_POINT('',#22096);
#6733=VERTEX_POINT('',#22098);
#6734=VERTEX_POINT('',#22100);
#6735=VERTEX_POINT('',#22102);
#6736=VERTEX_POINT('',#22104);
#6737=VERTEX_POINT('',#22106);
#6738=VERTEX_POINT('',#22110);
#6739=VERTEX_POINT('',#22111);
#6740=VERTEX_POINT('',#22113);
#6741=VERTEX_POINT('',#22115);
#6742=VERTEX_POINT('',#22117);
#6743=VERTEX_POINT('',#22119);
#6744=VERTEX_POINT('',#22121);
#6745=VERTEX_POINT('',#22123);
#6746=VERTEX_POINT('',#22125);
#6747=VERTEX_POINT('',#22147);
#6748=VERTEX_POINT('',#22149);
#6749=VERTEX_POINT('',#22153);
#6750=VERTEX_POINT('',#22154);
#6751=VERTEX_POINT('',#22156);
#6752=VERTEX_POINT('',#22158);
#6753=VERTEX_POINT('',#22162);
#6754=VERTEX_POINT('',#22164);
#6755=VERTEX_POINT('',#22168);
#6756=VERTEX_POINT('',#22170);
#6757=VERTEX_POINT('',#22174);
#6758=VERTEX_POINT('',#22176);
#6759=VERTEX_POINT('',#22180);
#6760=VERTEX_POINT('',#22182);
#6761=VERTEX_POINT('',#22191);
#6762=VERTEX_POINT('',#22193);
#6763=VERTEX_POINT('',#22197);
#6764=VERTEX_POINT('',#22198);
#6765=VERTEX_POINT('',#22200);
#6766=VERTEX_POINT('',#22202);
#6767=VERTEX_POINT('',#22204);
#6768=VERTEX_POINT('',#22206);
#6769=VERTEX_POINT('',#22210);
#6770=VERTEX_POINT('',#22211);
#6771=VERTEX_POINT('',#22213);
#6772=VERTEX_POINT('',#22215);
#6773=VERTEX_POINT('',#22217);
#6774=VERTEX_POINT('',#22219);
#6775=VERTEX_POINT('',#22235);
#6776=VERTEX_POINT('',#22237);
#6777=VERTEX_POINT('',#22241);
#6778=VERTEX_POINT('',#22242);
#6779=VERTEX_POINT('',#22244);
#6780=VERTEX_POINT('',#22246);
#6781=VERTEX_POINT('',#22250);
#6782=VERTEX_POINT('',#22252);
#6783=VERTEX_POINT('',#22256);
#6784=VERTEX_POINT('',#22258);
#6785=VERTEX_POINT('',#22262);
#6786=VERTEX_POINT('',#22264);
#6787=VERTEX_POINT('',#22268);
#6788=VERTEX_POINT('',#22270);
#6789=VERTEX_POINT('',#22279);
#6790=VERTEX_POINT('',#22281);
#6791=VERTEX_POINT('',#22285);
#6792=VERTEX_POINT('',#22286);
#6793=VERTEX_POINT('',#22288);
#6794=VERTEX_POINT('',#22290);
#6795=VERTEX_POINT('',#22292);
#6796=VERTEX_POINT('',#22294);
#6797=VERTEX_POINT('',#22298);
#6798=VERTEX_POINT('',#22299);
#6799=VERTEX_POINT('',#22301);
#6800=VERTEX_POINT('',#22303);
#6801=VERTEX_POINT('',#22305);
#6802=VERTEX_POINT('',#22307);
#6803=VERTEX_POINT('',#22323);
#6804=VERTEX_POINT('',#22324);
#6805=VERTEX_POINT('',#22326);
#6806=VERTEX_POINT('',#22328);
#6807=VERTEX_POINT('',#22332);
#6808=VERTEX_POINT('',#22333);
#6809=VERTEX_POINT('',#22335);
#6810=VERTEX_POINT('',#22337);
#6811=VERTEX_POINT('',#22341);
#6812=VERTEX_POINT('',#22342);
#6813=VERTEX_POINT('',#22344);
#6814=VERTEX_POINT('',#22346);
#6815=VERTEX_POINT('',#22350);
#6816=VERTEX_POINT('',#22351);
#6817=VERTEX_POINT('',#22353);
#6818=VERTEX_POINT('',#22355);
#6819=VERTEX_POINT('',#22359);
#6820=VERTEX_POINT('',#22361);
#6821=VERTEX_POINT('',#22365);
#6822=VERTEX_POINT('',#22367);
#6823=VERTEX_POINT('',#22371);
#6824=VERTEX_POINT('',#22372);
#6825=VERTEX_POINT('',#22374);
#6826=VERTEX_POINT('',#22376);
#6827=VERTEX_POINT('',#22378);
#6828=VERTEX_POINT('',#22380);
#6829=VERTEX_POINT('',#22382);
#6830=VERTEX_POINT('',#22384);
#6831=VERTEX_POINT('',#22386);
#6832=VERTEX_POINT('',#22390);
#6833=VERTEX_POINT('',#22392);
#6834=VERTEX_POINT('',#22394);
#6835=VERTEX_POINT('',#22396);
#6836=VERTEX_POINT('',#22398);
#6837=VERTEX_POINT('',#22400);
#6838=VERTEX_POINT('',#22405);
#6839=VERTEX_POINT('',#22425);
#6840=VERTEX_POINT('',#22429);
#6841=VERTEX_POINT('',#22439);
#6842=VERTEX_POINT('',#22441);
#6843=VERTEX_POINT('',#22445);
#6844=VERTEX_POINT('',#22446);
#6845=VERTEX_POINT('',#22448);
#6846=VERTEX_POINT('',#22450);
#6847=VERTEX_POINT('',#22452);
#6848=VERTEX_POINT('',#22454);
#6849=VERTEX_POINT('',#22458);
#6850=VERTEX_POINT('',#22459);
#6851=VERTEX_POINT('',#22461);
#6852=VERTEX_POINT('',#22463);
#6853=VERTEX_POINT('',#22465);
#6854=VERTEX_POINT('',#22467);
#6855=VERTEX_POINT('',#22483);
#6856=VERTEX_POINT('',#22485);
#6857=VERTEX_POINT('',#22489);
#6858=VERTEX_POINT('',#22490);
#6859=VERTEX_POINT('',#22492);
#6860=VERTEX_POINT('',#22494);
#6861=VERTEX_POINT('',#22496);
#6862=VERTEX_POINT('',#22498);
#6863=VERTEX_POINT('',#22502);
#6864=VERTEX_POINT('',#22503);
#6865=VERTEX_POINT('',#22505);
#6866=VERTEX_POINT('',#22507);
#6867=VERTEX_POINT('',#22509);
#6868=VERTEX_POINT('',#22511);
#8155=EDGE_CURVE('',#6693,#6694,#3871,.T.);
#8156=EDGE_CURVE('',#6695,#6693,#3872,.T.);
#8157=EDGE_CURVE('',#6696,#6695,#3873,.T.);
#8158=EDGE_CURVE('',#6697,#6696,#3874,.T.);
#8159=EDGE_CURVE('',#6698,#6697,#644,.T.);
#8160=EDGE_CURVE('',#6699,#6698,#3875,.T.);
#8161=EDGE_CURVE('',#6700,#6699,#645,.T.);
#8162=EDGE_CURVE('',#6701,#6700,#3876,.T.);
#8163=EDGE_CURVE('',#6694,#6701,#646,.T.);
#8164=EDGE_CURVE('',#6702,#6703,#3877,.T.);
#8165=EDGE_CURVE('',#6704,#6702,#3878,.T.);
#8166=EDGE_CURVE('',#6705,#6704,#647,.T.);
#8167=EDGE_CURVE('',#6706,#6705,#3879,.T.);
#8168=EDGE_CURVE('',#6707,#6706,#648,.T.);
#8169=EDGE_CURVE('',#6708,#6707,#3880,.T.);
#8170=EDGE_CURVE('',#6709,#6708,#649,.T.);
#8171=EDGE_CURVE('',#6710,#6709,#3881,.T.);
#8172=EDGE_CURVE('',#6703,#6710,#3882,.T.);
#8173=EDGE_CURVE('',#6695,#6703,#3883,.T.);
#8174=EDGE_CURVE('',#6693,#6702,#3884,.T.);
#8175=EDGE_CURVE('',#6696,#6710,#3885,.T.);
#8176=EDGE_CURVE('',#6697,#6709,#3886,.T.);
#8177=EDGE_CURVE('',#6698,#6708,#3887,.T.);
#8178=EDGE_CURVE('',#6699,#6707,#3888,.T.);
#8179=EDGE_CURVE('',#6700,#6706,#3889,.T.);
#8180=EDGE_CURVE('',#6701,#6705,#3890,.T.);
#8181=EDGE_CURVE('',#6694,#6704,#3891,.T.);
#8182=EDGE_CURVE('',#6711,#6712,#3892,.T.);
#8183=EDGE_CURVE('',#6713,#6711,#650,.T.);
#8184=EDGE_CURVE('',#6714,#6713,#3893,.T.);
#8185=EDGE_CURVE('',#6715,#6714,#651,.T.);
#8186=EDGE_CURVE('',#6716,#6715,#3894,.T.);
#8187=EDGE_CURVE('',#6717,#6716,#652,.T.);
#8188=EDGE_CURVE('',#6718,#6717,#3895,.T.);
#8189=EDGE_CURVE('',#6719,#6718,#3896,.T.);
#8190=EDGE_CURVE('',#6712,#6719,#3897,.T.);
#8191=EDGE_CURVE('',#6720,#6721,#3898,.T.);
#8192=EDGE_CURVE('',#6722,#6720,#3899,.T.);
#8193=EDGE_CURVE('',#6723,#6722,#3900,.T.);
#8194=EDGE_CURVE('',#6724,#6723,#653,.T.);
#8195=EDGE_CURVE('',#6725,#6724,#3901,.T.);
#8196=EDGE_CURVE('',#6726,#6725,#654,.T.);
#8197=EDGE_CURVE('',#6727,#6726,#3902,.T.);
#8198=EDGE_CURVE('',#6728,#6727,#655,.T.);
#8199=EDGE_CURVE('',#6721,#6728,#3903,.T.);
#8200=EDGE_CURVE('',#6721,#6712,#3904,.T.);
#8201=EDGE_CURVE('',#6720,#6719,#3905,.T.);
#8202=EDGE_CURVE('',#6722,#6718,#3906,.T.);
#8203=EDGE_CURVE('',#6723,#6717,#3907,.T.);
#8204=EDGE_CURVE('',#6724,#6716,#3908,.T.);
#8205=EDGE_CURVE('',#6725,#6715,#3909,.T.);
#8206=EDGE_CURVE('',#6726,#6714,#3910,.T.);
#8207=EDGE_CURVE('',#6727,#6713,#3911,.T.);
#8208=EDGE_CURVE('',#6728,#6711,#3912,.T.);
#8209=EDGE_CURVE('',#6729,#6730,#3913,.T.);
#8210=EDGE_CURVE('',#6731,#6729,#656,.T.);
#8211=EDGE_CURVE('',#6732,#6731,#3914,.T.);
#8212=EDGE_CURVE('',#6733,#6732,#657,.T.);
#8213=EDGE_CURVE('',#6734,#6733,#3915,.T.);
#8214=EDGE_CURVE('',#6735,#6734,#658,.T.);
#8215=EDGE_CURVE('',#6736,#6735,#3916,.T.);
#8216=EDGE_CURVE('',#6737,#6736,#3917,.T.);
#8217=EDGE_CURVE('',#6730,#6737,#3918,.T.);
#8218=EDGE_CURVE('',#6738,#6739,#3919,.T.);
#8219=EDGE_CURVE('',#6740,#6738,#3920,.T.);
#8220=EDGE_CURVE('',#6741,#6740,#3921,.T.);
#8221=EDGE_CURVE('',#6742,#6741,#659,.T.);
#8222=EDGE_CURVE('',#6743,#6742,#3922,.T.);
#8223=EDGE_CURVE('',#6744,#6743,#660,.T.);
#8224=EDGE_CURVE('',#6745,#6744,#3923,.T.);
#8225=EDGE_CURVE('',#6746,#6745,#661,.T.);
#8226=EDGE_CURVE('',#6739,#6746,#3924,.T.);
#8227=EDGE_CURVE('',#6739,#6730,#3925,.T.);
#8228=EDGE_CURVE('',#6738,#6737,#3926,.T.);
#8229=EDGE_CURVE('',#6740,#6736,#3927,.T.);
#8230=EDGE_CURVE('',#6741,#6735,#3928,.T.);
#8231=EDGE_CURVE('',#6742,#6734,#3929,.T.);
#8232=EDGE_CURVE('',#6743,#6733,#3930,.T.);
#8233=EDGE_CURVE('',#6744,#6732,#3931,.T.);
#8234=EDGE_CURVE('',#6745,#6731,#3932,.T.);
#8235=EDGE_CURVE('',#6746,#6729,#3933,.T.);
#8236=EDGE_CURVE('',#6747,#6747,#820,.T.);
#8237=EDGE_CURVE('',#6747,#6748,#3934,.T.);
#8238=EDGE_CURVE('',#6748,#6748,#821,.T.);
#8239=EDGE_CURVE('',#6749,#6750,#822,.T.);
#8240=EDGE_CURVE('',#6750,#6751,#3935,.T.);
#8241=EDGE_CURVE('',#6752,#6751,#823,.T.);
#8242=EDGE_CURVE('',#6749,#6752,#3936,.T.);
#8243=EDGE_CURVE('',#6753,#6752,#824,.T.);
#8244=EDGE_CURVE('',#6754,#6753,#3937,.T.);
#8245=EDGE_CURVE('',#6754,#6749,#825,.T.);
#8246=EDGE_CURVE('',#6755,#6753,#3938,.T.);
#8247=EDGE_CURVE('',#6756,#6755,#3939,.T.);
#8248=EDGE_CURVE('',#6756,#6754,#3940,.T.);
#8249=EDGE_CURVE('',#6757,#6755,#3941,.T.);
#8250=EDGE_CURVE('',#6758,#6757,#3942,.T.);
#8251=EDGE_CURVE('',#6758,#6756,#3943,.T.);
#8252=EDGE_CURVE('',#6759,#6757,#3944,.T.);
#8253=EDGE_CURVE('',#6760,#6759,#3945,.T.);
#8254=EDGE_CURVE('',#6760,#6758,#3946,.T.);
#8255=EDGE_CURVE('',#6751,#6759,#3947,.T.);
#8256=EDGE_CURVE('',#6750,#6760,#3948,.T.);
#8257=EDGE_CURVE('',#6761,#6761,#826,.T.);
#8258=EDGE_CURVE('',#6761,#6762,#3949,.T.);
#8259=EDGE_CURVE('',#6762,#6762,#827,.T.);
#8260=EDGE_CURVE('',#6763,#6764,#3950,.T.);
#8261=EDGE_CURVE('',#6764,#6765,#3951,.T.);
#8262=EDGE_CURVE('',#6765,#6766,#3952,.T.);
#8263=EDGE_CURVE('',#6766,#6767,#828,.T.);
#8264=EDGE_CURVE('',#6767,#6768,#3953,.T.);
#8265=EDGE_CURVE('',#6768,#6763,#3954,.T.);
#8266=EDGE_CURVE('',#6769,#6770,#3955,.T.);
#8267=EDGE_CURVE('',#6771,#6769,#3956,.T.);
#8268=EDGE_CURVE('',#6772,#6771,#3957,.T.);
#8269=EDGE_CURVE('',#6773,#6772,#829,.T.);
#8270=EDGE_CURVE('',#6774,#6773,#3958,.T.);
#8271=EDGE_CURVE('',#6770,#6774,#3959,.T.);
#8272=EDGE_CURVE('',#6764,#6770,#3960,.T.);
#8273=EDGE_CURVE('',#6763,#6769,#3961,.T.);
#8274=EDGE_CURVE('',#6765,#6774,#3962,.T.);
#8275=EDGE_CURVE('',#6766,#6773,#3963,.T.);
#8276=EDGE_CURVE('',#6767,#6772,#3964,.T.);
#8277=EDGE_CURVE('',#6768,#6771,#3965,.T.);
#8278=EDGE_CURVE('',#6775,#6775,#830,.T.);
#8279=EDGE_CURVE('',#6775,#6776,#3966,.T.);
#8280=EDGE_CURVE('',#6776,#6776,#831,.T.);
#8281=EDGE_CURVE('',#6777,#6778,#832,.T.);
#8282=EDGE_CURVE('',#6777,#6779,#3967,.T.);
#8283=EDGE_CURVE('',#6779,#6780,#833,.T.);
#8284=EDGE_CURVE('',#6778,#6780,#3968,.T.);
#8285=EDGE_CURVE('',#6781,#6779,#834,.T.);
#8286=EDGE_CURVE('',#6782,#6777,#835,.T.);
#8287=EDGE_CURVE('',#6782,#6781,#3969,.T.);
#8288=EDGE_CURVE('',#6783,#6781,#3970,.T.);
#8289=EDGE_CURVE('',#6784,#6782,#3971,.T.);
#8290=EDGE_CURVE('',#6784,#6783,#3972,.T.);
#8291=EDGE_CURVE('',#6785,#6783,#3973,.T.);
#8292=EDGE_CURVE('',#6786,#6784,#3974,.T.);
#8293=EDGE_CURVE('',#6786,#6785,#3975,.T.);
#8294=EDGE_CURVE('',#6787,#6785,#3976,.T.);
#8295=EDGE_CURVE('',#6788,#6786,#3977,.T.);
#8296=EDGE_CURVE('',#6788,#6787,#3978,.T.);
#8297=EDGE_CURVE('',#6780,#6787,#3979,.T.);
#8298=EDGE_CURVE('',#6778,#6788,#3980,.T.);
#8299=EDGE_CURVE('',#6789,#6789,#836,.T.);
#8300=EDGE_CURVE('',#6789,#6790,#3981,.T.);
#8301=EDGE_CURVE('',#6790,#6790,#837,.T.);
#8302=EDGE_CURVE('',#6791,#6792,#3982,.T.);
#8303=EDGE_CURVE('',#6793,#6791,#3983,.T.);
#8304=EDGE_CURVE('',#6794,#6793,#3984,.T.);
#8305=EDGE_CURVE('',#6795,#6794,#838,.T.);
#8306=EDGE_CURVE('',#6796,#6795,#3985,.T.);
#8307=EDGE_CURVE('',#6792,#6796,#3986,.T.);
#8308=EDGE_CURVE('',#6797,#6798,#3987,.T.);
#8309=EDGE_CURVE('',#6798,#6799,#3988,.T.);
#8310=EDGE_CURVE('',#6799,#6800,#3989,.T.);
#8311=EDGE_CURVE('',#6800,#6801,#839,.T.);
#8312=EDGE_CURVE('',#6801,#6802,#3990,.T.);
#8313=EDGE_CURVE('',#6802,#6797,#3991,.T.);
#8314=EDGE_CURVE('',#6791,#6797,#3992,.T.);
#8315=EDGE_CURVE('',#6792,#6798,#3993,.T.);
#8316=EDGE_CURVE('',#6796,#6799,#3994,.T.);
#8317=EDGE_CURVE('',#6795,#6800,#3995,.T.);
#8318=EDGE_CURVE('',#6794,#6801,#3996,.T.);
#8319=EDGE_CURVE('',#6793,#6802,#3997,.T.);
#8320=EDGE_CURVE('',#6803,#6804,#840,.T.);
#8321=EDGE_CURVE('',#6804,#6805,#3998,.T.);
#8322=EDGE_CURVE('',#6805,#6806,#841,.T.);
#8323=EDGE_CURVE('',#6803,#6806,#3999,.T.);
#8324=EDGE_CURVE('',#6807,#6808,#842,.T.);
#8325=EDGE_CURVE('',#6808,#6809,#4000,.T.);
#8326=EDGE_CURVE('',#6809,#6810,#843,.T.);
#8327=EDGE_CURVE('',#6807,#6810,#4001,.T.);
#8328=EDGE_CURVE('',#6811,#6812,#844,.T.);
#8329=EDGE_CURVE('',#6813,#6811,#4002,.T.);
#8330=EDGE_CURVE('',#6814,#6813,#845,.T.);
#8331=EDGE_CURVE('',#6814,#6812,#4003,.T.);
#8332=EDGE_CURVE('',#6815,#6816,#846,.T.);
#8333=EDGE_CURVE('',#6817,#6815,#4004,.T.);
#8334=EDGE_CURVE('',#6817,#6818,#662,.T.);
#8335=EDGE_CURVE('',#6818,#6816,#4005,.T.);
#8336=EDGE_CURVE('',#6819,#6811,#4006,.T.);
#8337=EDGE_CURVE('',#6820,#6819,#4007,.T.);
#8338=EDGE_CURVE('',#6813,#6820,#4008,.T.);
#8339=EDGE_CURVE('',#6821,#6815,#4009,.T.);
#8340=EDGE_CURVE('',#6822,#6821,#4010,.T.);
#8341=EDGE_CURVE('',#6822,#6817,#4011,.T.);
#8342=EDGE_CURVE('',#6823,#6824,#4012,.T.);
#8343=EDGE_CURVE('',#6825,#6823,#663,.T.);
#8344=EDGE_CURVE('',#6826,#6825,#4013,.T.);
#8345=EDGE_CURVE('',#6827,#6826,#664,.T.);
#8346=EDGE_CURVE('',#6828,#6827,#4014,.T.);
#8347=EDGE_CURVE('',#6829,#6828,#665,.T.);
#8348=EDGE_CURVE('',#6830,#6829,#4015,.T.);
#8349=EDGE_CURVE('',#6831,#6830,#4016,.T.);
#8350=EDGE_CURVE('',#6824,#6831,#4017,.T.);
#8351=EDGE_CURVE('',#6832,#6822,#4018,.T.);
#8352=EDGE_CURVE('',#6833,#6832,#4019,.T.);
#8353=EDGE_CURVE('',#6834,#6833,#4020,.T.);
#8354=EDGE_CURVE('',#6835,#6834,#666,.T.);
#8355=EDGE_CURVE('',#6836,#6835,#4021,.T.);
#8356=EDGE_CURVE('',#6837,#6836,#667,.T.);
#8357=EDGE_CURVE('',#6818,#6837,#4022,.T.);
#8358=EDGE_CURVE('',#6806,#6819,#4023,.T.);
#8359=EDGE_CURVE('',#6838,#6805,#4024,.T.);
#8360=EDGE_CURVE('',#6838,#6824,#4025,.T.);
#8361=EDGE_CURVE('',#6832,#6831,#4026,.T.);
#8362=EDGE_CURVE('',#6810,#6821,#4027,.T.);
#8363=EDGE_CURVE('',#6820,#6809,#4028,.T.);
#8364=EDGE_CURVE('',#6833,#6830,#4029,.T.);
#8365=EDGE_CURVE('',#6834,#6829,#4030,.T.);
#8366=EDGE_CURVE('',#6835,#6828,#4031,.T.);
#8367=EDGE_CURVE('',#6836,#6827,#4032,.T.);
#8368=EDGE_CURVE('',#6837,#6826,#4033,.T.);
#8369=EDGE_CURVE('',#6812,#6803,#4034,.T.);
#8370=EDGE_CURVE('',#6808,#6814,#4035,.T.);
#8371=EDGE_CURVE('',#6816,#6807,#4036,.T.);
#8372=EDGE_CURVE('',#6839,#6825,#4037,.T.);
#8373=EDGE_CURVE('',#6804,#6839,#4038,.T.);
#8374=EDGE_CURVE('',#6839,#6840,#847,.T.);
#8375=EDGE_CURVE('',#6840,#6823,#4039,.T.);
#8376=EDGE_CURVE('',#6840,#6838,#4040,.T.);
#8377=EDGE_CURVE('',#6841,#6841,#848,.T.);
#8378=EDGE_CURVE('',#6841,#6842,#4041,.T.);
#8379=EDGE_CURVE('',#6842,#6842,#849,.T.);
#8380=EDGE_CURVE('',#6843,#6844,#4042,.T.);
#8381=EDGE_CURVE('',#6845,#6843,#4043,.T.);
#8382=EDGE_CURVE('',#6846,#6845,#4044,.T.);
#8383=EDGE_CURVE('',#6847,#6846,#850,.T.);
#8384=EDGE_CURVE('',#6848,#6847,#4045,.T.);
#8385=EDGE_CURVE('',#6844,#6848,#4046,.T.);
#8386=EDGE_CURVE('',#6849,#6850,#4047,.T.);
#8387=EDGE_CURVE('',#6850,#6851,#4048,.T.);
#8388=EDGE_CURVE('',#6851,#6852,#4049,.T.);
#8389=EDGE_CURVE('',#6852,#6853,#851,.T.);
#8390=EDGE_CURVE('',#6853,#6854,#4050,.T.);
#8391=EDGE_CURVE('',#6854,#6849,#4051,.T.);
#8392=EDGE_CURVE('',#6843,#6849,#4052,.T.);
#8393=EDGE_CURVE('',#6844,#6850,#4053,.T.);
#8394=EDGE_CURVE('',#6848,#6851,#4054,.T.);
#8395=EDGE_CURVE('',#6847,#6852,#4055,.T.);
#8396=EDGE_CURVE('',#6846,#6853,#4056,.T.);
#8397=EDGE_CURVE('',#6845,#6854,#4057,.T.);
#8398=EDGE_CURVE('',#6855,#6855,#852,.T.);
#8399=EDGE_CURVE('',#6855,#6856,#4058,.T.);
#8400=EDGE_CURVE('',#6856,#6856,#853,.T.);
#8401=EDGE_CURVE('',#6857,#6858,#4059,.T.);
#8402=EDGE_CURVE('',#6858,#6859,#4060,.T.);
#8403=EDGE_CURVE('',#6859,#6860,#4061,.T.);
#8404=EDGE_CURVE('',#6860,#6861,#854,.T.);
#8405=EDGE_CURVE('',#6861,#6862,#4062,.T.);
#8406=EDGE_CURVE('',#6862,#6857,#4063,.T.);
#8407=EDGE_CURVE('',#6863,#6864,#4064,.T.);
#8408=EDGE_CURVE('',#6865,#6863,#4065,.T.);
#8409=EDGE_CURVE('',#6866,#6865,#4066,.T.);
#8410=EDGE_CURVE('',#6867,#6866,#855,.T.);
#8411=EDGE_CURVE('',#6868,#6867,#4067,.T.);
#8412=EDGE_CURVE('',#6864,#6868,#4068,.T.);
#8413=EDGE_CURVE('',#6858,#6864,#4069,.T.);
#8414=EDGE_CURVE('',#6857,#6863,#4070,.T.);
#8415=EDGE_CURVE('',#6859,#6868,#4071,.T.);
#8416=EDGE_CURVE('',#6860,#6867,#4072,.T.);
#8417=EDGE_CURVE('',#6861,#6866,#4073,.T.);
#8418=EDGE_CURVE('',#6862,#6865,#4074,.T.);
#10543=ORIENTED_EDGE('',*,*,#8155,.F.);
#10544=ORIENTED_EDGE('',*,*,#8156,.F.);
#10545=ORIENTED_EDGE('',*,*,#8157,.F.);
#10546=ORIENTED_EDGE('',*,*,#8158,.F.);
#10547=ORIENTED_EDGE('',*,*,#8159,.F.);
#10548=ORIENTED_EDGE('',*,*,#8160,.F.);
#10549=ORIENTED_EDGE('',*,*,#8161,.F.);
#10550=ORIENTED_EDGE('',*,*,#8162,.F.);
#10551=ORIENTED_EDGE('',*,*,#8163,.F.);
#10552=ORIENTED_EDGE('',*,*,#8164,.F.);
#10553=ORIENTED_EDGE('',*,*,#8165,.F.);
#10554=ORIENTED_EDGE('',*,*,#8166,.F.);
#10555=ORIENTED_EDGE('',*,*,#8167,.F.);
#10556=ORIENTED_EDGE('',*,*,#8168,.F.);
#10557=ORIENTED_EDGE('',*,*,#8169,.F.);
#10558=ORIENTED_EDGE('',*,*,#8170,.F.);
#10559=ORIENTED_EDGE('',*,*,#8171,.F.);
#10560=ORIENTED_EDGE('',*,*,#8172,.F.);
#10561=ORIENTED_EDGE('',*,*,#8173,.F.);
#10562=ORIENTED_EDGE('',*,*,#8156,.T.);
#10563=ORIENTED_EDGE('',*,*,#8174,.T.);
#10564=ORIENTED_EDGE('',*,*,#8164,.T.);
#10565=ORIENTED_EDGE('',*,*,#8175,.F.);
#10566=ORIENTED_EDGE('',*,*,#8157,.T.);
#10567=ORIENTED_EDGE('',*,*,#8173,.T.);
#10568=ORIENTED_EDGE('',*,*,#8172,.T.);
#10569=ORIENTED_EDGE('',*,*,#8176,.F.);
#10570=ORIENTED_EDGE('',*,*,#8158,.T.);
#10571=ORIENTED_EDGE('',*,*,#8175,.T.);
#10572=ORIENTED_EDGE('',*,*,#8171,.T.);
#10573=ORIENTED_EDGE('',*,*,#8177,.F.);
#10574=ORIENTED_EDGE('',*,*,#8159,.T.);
#10575=ORIENTED_EDGE('',*,*,#8176,.T.);
#10576=ORIENTED_EDGE('',*,*,#8170,.T.);
#10577=ORIENTED_EDGE('',*,*,#8178,.F.);
#10578=ORIENTED_EDGE('',*,*,#8160,.T.);
#10579=ORIENTED_EDGE('',*,*,#8177,.T.);
#10580=ORIENTED_EDGE('',*,*,#8169,.T.);
#10581=ORIENTED_EDGE('',*,*,#8179,.F.);
#10582=ORIENTED_EDGE('',*,*,#8161,.T.);
#10583=ORIENTED_EDGE('',*,*,#8178,.T.);
#10584=ORIENTED_EDGE('',*,*,#8168,.T.);
#10585=ORIENTED_EDGE('',*,*,#8180,.F.);
#10586=ORIENTED_EDGE('',*,*,#8162,.T.);
#10587=ORIENTED_EDGE('',*,*,#8179,.T.);
#10588=ORIENTED_EDGE('',*,*,#8167,.T.);
#10589=ORIENTED_EDGE('',*,*,#8181,.F.);
#10590=ORIENTED_EDGE('',*,*,#8163,.T.);
#10591=ORIENTED_EDGE('',*,*,#8180,.T.);
#10592=ORIENTED_EDGE('',*,*,#8166,.T.);
#10593=ORIENTED_EDGE('',*,*,#8174,.F.);
#10594=ORIENTED_EDGE('',*,*,#8155,.T.);
#10595=ORIENTED_EDGE('',*,*,#8181,.T.);
#10596=ORIENTED_EDGE('',*,*,#8165,.T.);
#10597=ORIENTED_EDGE('',*,*,#8182,.F.);
#10598=ORIENTED_EDGE('',*,*,#8183,.F.);
#10599=ORIENTED_EDGE('',*,*,#8184,.F.);
#10600=ORIENTED_EDGE('',*,*,#8185,.F.);
#10601=ORIENTED_EDGE('',*,*,#8186,.F.);
#10602=ORIENTED_EDGE('',*,*,#8187,.F.);
#10603=ORIENTED_EDGE('',*,*,#8188,.F.);
#10604=ORIENTED_EDGE('',*,*,#8189,.F.);
#10605=ORIENTED_EDGE('',*,*,#8190,.F.);
#10606=ORIENTED_EDGE('',*,*,#8191,.F.);
#10607=ORIENTED_EDGE('',*,*,#8192,.F.);
#10608=ORIENTED_EDGE('',*,*,#8193,.F.);
#10609=ORIENTED_EDGE('',*,*,#8194,.F.);
#10610=ORIENTED_EDGE('',*,*,#8195,.F.);
#10611=ORIENTED_EDGE('',*,*,#8196,.F.);
#10612=ORIENTED_EDGE('',*,*,#8197,.F.);
#10613=ORIENTED_EDGE('',*,*,#8198,.F.);
#10614=ORIENTED_EDGE('',*,*,#8199,.F.);
#10615=ORIENTED_EDGE('',*,*,#8200,.T.);
#10616=ORIENTED_EDGE('',*,*,#8190,.T.);
#10617=ORIENTED_EDGE('',*,*,#8201,.F.);
#10618=ORIENTED_EDGE('',*,*,#8191,.T.);
#10619=ORIENTED_EDGE('',*,*,#8201,.T.);
#10620=ORIENTED_EDGE('',*,*,#8189,.T.);
#10621=ORIENTED_EDGE('',*,*,#8202,.F.);
#10622=ORIENTED_EDGE('',*,*,#8192,.T.);
#10623=ORIENTED_EDGE('',*,*,#8202,.T.);
#10624=ORIENTED_EDGE('',*,*,#8188,.T.);
#10625=ORIENTED_EDGE('',*,*,#8203,.F.);
#10626=ORIENTED_EDGE('',*,*,#8193,.T.);
#10627=ORIENTED_EDGE('',*,*,#8203,.T.);
#10628=ORIENTED_EDGE('',*,*,#8187,.T.);
#10629=ORIENTED_EDGE('',*,*,#8204,.F.);
#10630=ORIENTED_EDGE('',*,*,#8194,.T.);
#10631=ORIENTED_EDGE('',*,*,#8204,.T.);
#10632=ORIENTED_EDGE('',*,*,#8186,.T.);
#10633=ORIENTED_EDGE('',*,*,#8205,.F.);
#10634=ORIENTED_EDGE('',*,*,#8195,.T.);
#10635=ORIENTED_EDGE('',*,*,#8205,.T.);
#10636=ORIENTED_EDGE('',*,*,#8185,.T.);
#10637=ORIENTED_EDGE('',*,*,#8206,.F.);
#10638=ORIENTED_EDGE('',*,*,#8196,.T.);
#10639=ORIENTED_EDGE('',*,*,#8206,.T.);
#10640=ORIENTED_EDGE('',*,*,#8184,.T.);
#10641=ORIENTED_EDGE('',*,*,#8207,.F.);
#10642=ORIENTED_EDGE('',*,*,#8197,.T.);
#10643=ORIENTED_EDGE('',*,*,#8207,.T.);
#10644=ORIENTED_EDGE('',*,*,#8183,.T.);
#10645=ORIENTED_EDGE('',*,*,#8208,.F.);
#10646=ORIENTED_EDGE('',*,*,#8198,.T.);
#10647=ORIENTED_EDGE('',*,*,#8208,.T.);
#10648=ORIENTED_EDGE('',*,*,#8182,.T.);
#10649=ORIENTED_EDGE('',*,*,#8200,.F.);
#10650=ORIENTED_EDGE('',*,*,#8199,.T.);
#10651=ORIENTED_EDGE('',*,*,#8209,.F.);
#10652=ORIENTED_EDGE('',*,*,#8210,.F.);
#10653=ORIENTED_EDGE('',*,*,#8211,.F.);
#10654=ORIENTED_EDGE('',*,*,#8212,.F.);
#10655=ORIENTED_EDGE('',*,*,#8213,.F.);
#10656=ORIENTED_EDGE('',*,*,#8214,.F.);
#10657=ORIENTED_EDGE('',*,*,#8215,.F.);
#10658=ORIENTED_EDGE('',*,*,#8216,.F.);
#10659=ORIENTED_EDGE('',*,*,#8217,.F.);
#10660=ORIENTED_EDGE('',*,*,#8218,.F.);
#10661=ORIENTED_EDGE('',*,*,#8219,.F.);
#10662=ORIENTED_EDGE('',*,*,#8220,.F.);
#10663=ORIENTED_EDGE('',*,*,#8221,.F.);
#10664=ORIENTED_EDGE('',*,*,#8222,.F.);
#10665=ORIENTED_EDGE('',*,*,#8223,.F.);
#10666=ORIENTED_EDGE('',*,*,#8224,.F.);
#10667=ORIENTED_EDGE('',*,*,#8225,.F.);
#10668=ORIENTED_EDGE('',*,*,#8226,.F.);
#10669=ORIENTED_EDGE('',*,*,#8227,.T.);
#10670=ORIENTED_EDGE('',*,*,#8217,.T.);
#10671=ORIENTED_EDGE('',*,*,#8228,.F.);
#10672=ORIENTED_EDGE('',*,*,#8218,.T.);
#10673=ORIENTED_EDGE('',*,*,#8228,.T.);
#10674=ORIENTED_EDGE('',*,*,#8216,.T.);
#10675=ORIENTED_EDGE('',*,*,#8229,.F.);
#10676=ORIENTED_EDGE('',*,*,#8219,.T.);
#10677=ORIENTED_EDGE('',*,*,#8229,.T.);
#10678=ORIENTED_EDGE('',*,*,#8215,.T.);
#10679=ORIENTED_EDGE('',*,*,#8230,.F.);
#10680=ORIENTED_EDGE('',*,*,#8220,.T.);
#10681=ORIENTED_EDGE('',*,*,#8230,.T.);
#10682=ORIENTED_EDGE('',*,*,#8214,.T.);
#10683=ORIENTED_EDGE('',*,*,#8231,.F.);
#10684=ORIENTED_EDGE('',*,*,#8221,.T.);
#10685=ORIENTED_EDGE('',*,*,#8231,.T.);
#10686=ORIENTED_EDGE('',*,*,#8213,.T.);
#10687=ORIENTED_EDGE('',*,*,#8232,.F.);
#10688=ORIENTED_EDGE('',*,*,#8222,.T.);
#10689=ORIENTED_EDGE('',*,*,#8232,.T.);
#10690=ORIENTED_EDGE('',*,*,#8212,.T.);
#10691=ORIENTED_EDGE('',*,*,#8233,.F.);
#10692=ORIENTED_EDGE('',*,*,#8223,.T.);
#10693=ORIENTED_EDGE('',*,*,#8233,.T.);
#10694=ORIENTED_EDGE('',*,*,#8211,.T.);
#10695=ORIENTED_EDGE('',*,*,#8234,.F.);
#10696=ORIENTED_EDGE('',*,*,#8224,.T.);
#10697=ORIENTED_EDGE('',*,*,#8234,.T.);
#10698=ORIENTED_EDGE('',*,*,#8210,.T.);
#10699=ORIENTED_EDGE('',*,*,#8235,.F.);
#10700=ORIENTED_EDGE('',*,*,#8225,.T.);
#10701=ORIENTED_EDGE('',*,*,#8235,.T.);
#10702=ORIENTED_EDGE('',*,*,#8209,.T.);
#10703=ORIENTED_EDGE('',*,*,#8227,.F.);
#10704=ORIENTED_EDGE('',*,*,#8226,.T.);
#10705=ORIENTED_EDGE('',*,*,#8236,.F.);
#10706=ORIENTED_EDGE('',*,*,#8237,.T.);
#10707=ORIENTED_EDGE('',*,*,#8238,.T.);
#10708=ORIENTED_EDGE('',*,*,#8237,.F.);
#10709=ORIENTED_EDGE('',*,*,#8239,.T.);
#10710=ORIENTED_EDGE('',*,*,#8240,.T.);
#10711=ORIENTED_EDGE('',*,*,#8241,.F.);
#10712=ORIENTED_EDGE('',*,*,#8242,.F.);
#10713=ORIENTED_EDGE('',*,*,#8243,.F.);
#10714=ORIENTED_EDGE('',*,*,#8244,.F.);
#10715=ORIENTED_EDGE('',*,*,#8245,.T.);
#10716=ORIENTED_EDGE('',*,*,#8242,.T.);
#10717=ORIENTED_EDGE('',*,*,#8246,.F.);
#10718=ORIENTED_EDGE('',*,*,#8247,.F.);
#10719=ORIENTED_EDGE('',*,*,#8248,.T.);
#10720=ORIENTED_EDGE('',*,*,#8244,.T.);
#10721=ORIENTED_EDGE('',*,*,#8249,.F.);
#10722=ORIENTED_EDGE('',*,*,#8250,.F.);
#10723=ORIENTED_EDGE('',*,*,#8251,.T.);
#10724=ORIENTED_EDGE('',*,*,#8247,.T.);
#10725=ORIENTED_EDGE('',*,*,#8252,.F.);
#10726=ORIENTED_EDGE('',*,*,#8253,.F.);
#10727=ORIENTED_EDGE('',*,*,#8254,.T.);
#10728=ORIENTED_EDGE('',*,*,#8250,.T.);
#10729=ORIENTED_EDGE('',*,*,#8255,.F.);
#10730=ORIENTED_EDGE('',*,*,#8240,.F.);
#10731=ORIENTED_EDGE('',*,*,#8256,.T.);
#10732=ORIENTED_EDGE('',*,*,#8253,.T.);
#10733=ORIENTED_EDGE('',*,*,#8239,.F.);
#10734=ORIENTED_EDGE('',*,*,#8245,.F.);
#10735=ORIENTED_EDGE('',*,*,#8248,.F.);
#10736=ORIENTED_EDGE('',*,*,#8251,.F.);
#10737=ORIENTED_EDGE('',*,*,#8254,.F.);
#10738=ORIENTED_EDGE('',*,*,#8256,.F.);
#10739=ORIENTED_EDGE('',*,*,#8236,.T.);
#10740=ORIENTED_EDGE('',*,*,#8241,.T.);
#10741=ORIENTED_EDGE('',*,*,#8255,.T.);
#10742=ORIENTED_EDGE('',*,*,#8252,.T.);
#10743=ORIENTED_EDGE('',*,*,#8249,.T.);
#10744=ORIENTED_EDGE('',*,*,#8246,.T.);
#10745=ORIENTED_EDGE('',*,*,#8243,.T.);
#10746=ORIENTED_EDGE('',*,*,#8238,.F.);
#10747=ORIENTED_EDGE('',*,*,#8257,.T.);
#10748=ORIENTED_EDGE('',*,*,#8258,.T.);
#10749=ORIENTED_EDGE('',*,*,#8259,.F.);
#10750=ORIENTED_EDGE('',*,*,#8258,.F.);
#10751=ORIENTED_EDGE('',*,*,#8260,.T.);
#10752=ORIENTED_EDGE('',*,*,#8261,.T.);
#10753=ORIENTED_EDGE('',*,*,#8262,.T.);
#10754=ORIENTED_EDGE('',*,*,#8263,.T.);
#10755=ORIENTED_EDGE('',*,*,#8264,.T.);
#10756=ORIENTED_EDGE('',*,*,#8265,.T.);
#10757=ORIENTED_EDGE('',*,*,#8257,.F.);
#10758=ORIENTED_EDGE('',*,*,#8266,.F.);
#10759=ORIENTED_EDGE('',*,*,#8267,.F.);
#10760=ORIENTED_EDGE('',*,*,#8268,.F.);
#10761=ORIENTED_EDGE('',*,*,#8269,.F.);
#10762=ORIENTED_EDGE('',*,*,#8270,.F.);
#10763=ORIENTED_EDGE('',*,*,#8271,.F.);
#10764=ORIENTED_EDGE('',*,*,#8259,.T.);
#10765=ORIENTED_EDGE('',*,*,#8266,.T.);
#10766=ORIENTED_EDGE('',*,*,#8272,.F.);
#10767=ORIENTED_EDGE('',*,*,#8260,.F.);
#10768=ORIENTED_EDGE('',*,*,#8273,.T.);
#10769=ORIENTED_EDGE('',*,*,#8271,.T.);
#10770=ORIENTED_EDGE('',*,*,#8274,.F.);
#10771=ORIENTED_EDGE('',*,*,#8261,.F.);
#10772=ORIENTED_EDGE('',*,*,#8272,.T.);
#10773=ORIENTED_EDGE('',*,*,#8270,.T.);
#10774=ORIENTED_EDGE('',*,*,#8275,.F.);
#10775=ORIENTED_EDGE('',*,*,#8262,.F.);
#10776=ORIENTED_EDGE('',*,*,#8274,.T.);
#10777=ORIENTED_EDGE('',*,*,#8269,.T.);
#10778=ORIENTED_EDGE('',*,*,#8276,.F.);
#10779=ORIENTED_EDGE('',*,*,#8263,.F.);
#10780=ORIENTED_EDGE('',*,*,#8275,.T.);
#10781=ORIENTED_EDGE('',*,*,#8268,.T.);
#10782=ORIENTED_EDGE('',*,*,#8277,.F.);
#10783=ORIENTED_EDGE('',*,*,#8264,.F.);
#10784=ORIENTED_EDGE('',*,*,#8276,.T.);
#10785=ORIENTED_EDGE('',*,*,#8267,.T.);
#10786=ORIENTED_EDGE('',*,*,#8273,.F.);
#10787=ORIENTED_EDGE('',*,*,#8265,.F.);
#10788=ORIENTED_EDGE('',*,*,#8277,.T.);
#10789=ORIENTED_EDGE('',*,*,#8278,.T.);
#10790=ORIENTED_EDGE('',*,*,#8279,.T.);
#10791=ORIENTED_EDGE('',*,*,#8280,.F.);
#10792=ORIENTED_EDGE('',*,*,#8279,.F.);
#10793=ORIENTED_EDGE('',*,*,#8281,.F.);
#10794=ORIENTED_EDGE('',*,*,#8282,.T.);
#10795=ORIENTED_EDGE('',*,*,#8283,.T.);
#10796=ORIENTED_EDGE('',*,*,#8284,.F.);
#10797=ORIENTED_EDGE('',*,*,#8285,.T.);
#10798=ORIENTED_EDGE('',*,*,#8282,.F.);
#10799=ORIENTED_EDGE('',*,*,#8286,.F.);
#10800=ORIENTED_EDGE('',*,*,#8287,.T.);
#10801=ORIENTED_EDGE('',*,*,#8288,.T.);
#10802=ORIENTED_EDGE('',*,*,#8287,.F.);
#10803=ORIENTED_EDGE('',*,*,#8289,.F.);
#10804=ORIENTED_EDGE('',*,*,#8290,.T.);
#10805=ORIENTED_EDGE('',*,*,#8291,.T.);
#10806=ORIENTED_EDGE('',*,*,#8290,.F.);
#10807=ORIENTED_EDGE('',*,*,#8292,.F.);
#10808=ORIENTED_EDGE('',*,*,#8293,.T.);
#10809=ORIENTED_EDGE('',*,*,#8294,.T.);
#10810=ORIENTED_EDGE('',*,*,#8293,.F.);
#10811=ORIENTED_EDGE('',*,*,#8295,.F.);
#10812=ORIENTED_EDGE('',*,*,#8296,.T.);
#10813=ORIENTED_EDGE('',*,*,#8297,.T.);
#10814=ORIENTED_EDGE('',*,*,#8296,.F.);
#10815=ORIENTED_EDGE('',*,*,#8298,.F.);
#10816=ORIENTED_EDGE('',*,*,#8284,.T.);
#10817=ORIENTED_EDGE('',*,*,#8281,.T.);
#10818=ORIENTED_EDGE('',*,*,#8298,.T.);
#10819=ORIENTED_EDGE('',*,*,#8295,.T.);
#10820=ORIENTED_EDGE('',*,*,#8292,.T.);
#10821=ORIENTED_EDGE('',*,*,#8289,.T.);
#10822=ORIENTED_EDGE('',*,*,#8286,.T.);
#10823=ORIENTED_EDGE('',*,*,#8278,.F.);
#10824=ORIENTED_EDGE('',*,*,#8283,.F.);
#10825=ORIENTED_EDGE('',*,*,#8285,.F.);
#10826=ORIENTED_EDGE('',*,*,#8288,.F.);
#10827=ORIENTED_EDGE('',*,*,#8291,.F.);
#10828=ORIENTED_EDGE('',*,*,#8294,.F.);
#10829=ORIENTED_EDGE('',*,*,#8297,.F.);
#10830=ORIENTED_EDGE('',*,*,#8280,.T.);
#10831=ORIENTED_EDGE('',*,*,#8299,.F.);
#10832=ORIENTED_EDGE('',*,*,#8300,.T.);
#10833=ORIENTED_EDGE('',*,*,#8301,.T.);
#10834=ORIENTED_EDGE('',*,*,#8300,.F.);
#10835=ORIENTED_EDGE('',*,*,#8302,.F.);
#10836=ORIENTED_EDGE('',*,*,#8303,.F.);
#10837=ORIENTED_EDGE('',*,*,#8304,.F.);
#10838=ORIENTED_EDGE('',*,*,#8305,.F.);
#10839=ORIENTED_EDGE('',*,*,#8306,.F.);
#10840=ORIENTED_EDGE('',*,*,#8307,.F.);
#10841=ORIENTED_EDGE('',*,*,#8299,.T.);
#10842=ORIENTED_EDGE('',*,*,#8308,.T.);
#10843=ORIENTED_EDGE('',*,*,#8309,.T.);
#10844=ORIENTED_EDGE('',*,*,#8310,.T.);
#10845=ORIENTED_EDGE('',*,*,#8311,.T.);
#10846=ORIENTED_EDGE('',*,*,#8312,.T.);
#10847=ORIENTED_EDGE('',*,*,#8313,.T.);
#10848=ORIENTED_EDGE('',*,*,#8301,.F.);
#10849=ORIENTED_EDGE('',*,*,#8308,.F.);
#10850=ORIENTED_EDGE('',*,*,#8314,.F.);
#10851=ORIENTED_EDGE('',*,*,#8302,.T.);
#10852=ORIENTED_EDGE('',*,*,#8315,.T.);
#10853=ORIENTED_EDGE('',*,*,#8309,.F.);
#10854=ORIENTED_EDGE('',*,*,#8315,.F.);
#10855=ORIENTED_EDGE('',*,*,#8307,.T.);
#10856=ORIENTED_EDGE('',*,*,#8316,.T.);
#10857=ORIENTED_EDGE('',*,*,#8310,.F.);
#10858=ORIENTED_EDGE('',*,*,#8316,.F.);
#10859=ORIENTED_EDGE('',*,*,#8306,.T.);
#10860=ORIENTED_EDGE('',*,*,#8317,.T.);
#10861=ORIENTED_EDGE('',*,*,#8311,.F.);
#10862=ORIENTED_EDGE('',*,*,#8317,.F.);
#10863=ORIENTED_EDGE('',*,*,#8305,.T.);
#10864=ORIENTED_EDGE('',*,*,#8318,.T.);
#10865=ORIENTED_EDGE('',*,*,#8312,.F.);
#10866=ORIENTED_EDGE('',*,*,#8318,.F.);
#10867=ORIENTED_EDGE('',*,*,#8304,.T.);
#10868=ORIENTED_EDGE('',*,*,#8319,.T.);
#10869=ORIENTED_EDGE('',*,*,#8313,.F.);
#10870=ORIENTED_EDGE('',*,*,#8319,.F.);
#10871=ORIENTED_EDGE('',*,*,#8303,.T.);
#10872=ORIENTED_EDGE('',*,*,#8314,.T.);
#10873=ORIENTED_EDGE('',*,*,#8320,.T.);
#10874=ORIENTED_EDGE('',*,*,#8321,.T.);
#10875=ORIENTED_EDGE('',*,*,#8322,.T.);
#10876=ORIENTED_EDGE('',*,*,#8323,.F.);
#10877=ORIENTED_EDGE('',*,*,#8324,.T.);
#10878=ORIENTED_EDGE('',*,*,#8325,.T.);
#10879=ORIENTED_EDGE('',*,*,#8326,.T.);
#10880=ORIENTED_EDGE('',*,*,#8327,.F.);
#10881=ORIENTED_EDGE('',*,*,#8328,.F.);
#10882=ORIENTED_EDGE('',*,*,#8329,.F.);
#10883=ORIENTED_EDGE('',*,*,#8330,.F.);
#10884=ORIENTED_EDGE('',*,*,#8331,.T.);
#10885=ORIENTED_EDGE('',*,*,#8332,.F.);
#10886=ORIENTED_EDGE('',*,*,#8333,.F.);
#10887=ORIENTED_EDGE('',*,*,#8334,.T.);
#10888=ORIENTED_EDGE('',*,*,#8335,.T.);
#10889=ORIENTED_EDGE('',*,*,#8336,.F.);
#10890=ORIENTED_EDGE('',*,*,#8337,.F.);
#10891=ORIENTED_EDGE('',*,*,#8338,.F.);
#10892=ORIENTED_EDGE('',*,*,#8329,.T.);
#10893=ORIENTED_EDGE('',*,*,#8339,.F.);
#10894=ORIENTED_EDGE('',*,*,#8340,.F.);
#10895=ORIENTED_EDGE('',*,*,#8341,.T.);
#10896=ORIENTED_EDGE('',*,*,#8333,.T.);
#10897=ORIENTED_EDGE('',*,*,#8342,.F.);
#10898=ORIENTED_EDGE('',*,*,#8343,.F.);
#10899=ORIENTED_EDGE('',*,*,#8344,.F.);
#10900=ORIENTED_EDGE('',*,*,#8345,.F.);
#10901=ORIENTED_EDGE('',*,*,#8346,.F.);
#10902=ORIENTED_EDGE('',*,*,#8347,.F.);
#10903=ORIENTED_EDGE('',*,*,#8348,.F.);
#10904=ORIENTED_EDGE('',*,*,#8349,.F.);
#10905=ORIENTED_EDGE('',*,*,#8350,.F.);
#10906=ORIENTED_EDGE('',*,*,#8351,.F.);
#10907=ORIENTED_EDGE('',*,*,#8352,.F.);
#10908=ORIENTED_EDGE('',*,*,#8353,.F.);
#10909=ORIENTED_EDGE('',*,*,#8354,.F.);
#10910=ORIENTED_EDGE('',*,*,#8355,.F.);
#10911=ORIENTED_EDGE('',*,*,#8356,.F.);
#10912=ORIENTED_EDGE('',*,*,#8357,.F.);
#10913=ORIENTED_EDGE('',*,*,#8334,.F.);
#10914=ORIENTED_EDGE('',*,*,#8341,.F.);
#10915=ORIENTED_EDGE('',*,*,#8358,.F.);
#10916=ORIENTED_EDGE('',*,*,#8322,.F.);
#10917=ORIENTED_EDGE('',*,*,#8359,.F.);
#10918=ORIENTED_EDGE('',*,*,#8360,.T.);
#10919=ORIENTED_EDGE('',*,*,#8350,.T.);
#10920=ORIENTED_EDGE('',*,*,#8361,.F.);
#10921=ORIENTED_EDGE('',*,*,#8351,.T.);
#10922=ORIENTED_EDGE('',*,*,#8340,.T.);
#10923=ORIENTED_EDGE('',*,*,#8362,.F.);
#10924=ORIENTED_EDGE('',*,*,#8326,.F.);
#10925=ORIENTED_EDGE('',*,*,#8363,.F.);
#10926=ORIENTED_EDGE('',*,*,#8337,.T.);
#10927=ORIENTED_EDGE('',*,*,#8361,.T.);
#10928=ORIENTED_EDGE('',*,*,#8349,.T.);
#10929=ORIENTED_EDGE('',*,*,#8364,.F.);
#10930=ORIENTED_EDGE('',*,*,#8352,.T.);
#10931=ORIENTED_EDGE('',*,*,#8364,.T.);
#10932=ORIENTED_EDGE('',*,*,#8348,.T.);
#10933=ORIENTED_EDGE('',*,*,#8365,.F.);
#10934=ORIENTED_EDGE('',*,*,#8353,.T.);
#10935=ORIENTED_EDGE('',*,*,#8365,.T.);
#10936=ORIENTED_EDGE('',*,*,#8347,.T.);
#10937=ORIENTED_EDGE('',*,*,#8366,.F.);
#10938=ORIENTED_EDGE('',*,*,#8354,.T.);
#10939=ORIENTED_EDGE('',*,*,#8366,.T.);
#10940=ORIENTED_EDGE('',*,*,#8346,.T.);
#10941=ORIENTED_EDGE('',*,*,#8367,.F.);
#10942=ORIENTED_EDGE('',*,*,#8355,.T.);
#10943=ORIENTED_EDGE('',*,*,#8367,.T.);
#10944=ORIENTED_EDGE('',*,*,#8345,.T.);
#10945=ORIENTED_EDGE('',*,*,#8368,.F.);
#10946=ORIENTED_EDGE('',*,*,#8356,.T.);
#10947=ORIENTED_EDGE('',*,*,#8369,.F.);
#10948=ORIENTED_EDGE('',*,*,#8331,.F.);
#10949=ORIENTED_EDGE('',*,*,#8370,.F.);
#10950=ORIENTED_EDGE('',*,*,#8324,.F.);
#10951=ORIENTED_EDGE('',*,*,#8371,.F.);
#10952=ORIENTED_EDGE('',*,*,#8335,.F.);
#10953=ORIENTED_EDGE('',*,*,#8357,.T.);
#10954=ORIENTED_EDGE('',*,*,#8368,.T.);
#10955=ORIENTED_EDGE('',*,*,#8344,.T.);
#10956=ORIENTED_EDGE('',*,*,#8372,.F.);
#10957=ORIENTED_EDGE('',*,*,#8373,.F.);
#10958=ORIENTED_EDGE('',*,*,#8320,.F.);
#10959=ORIENTED_EDGE('',*,*,#8374,.F.);
#10960=ORIENTED_EDGE('',*,*,#8372,.T.);
#10961=ORIENTED_EDGE('',*,*,#8343,.T.);
#10962=ORIENTED_EDGE('',*,*,#8375,.F.);
#10963=ORIENTED_EDGE('',*,*,#8376,.F.);
#10964=ORIENTED_EDGE('',*,*,#8375,.T.);
#10965=ORIENTED_EDGE('',*,*,#8342,.T.);
#10966=ORIENTED_EDGE('',*,*,#8360,.F.);
#10967=ORIENTED_EDGE('',*,*,#8371,.T.);
#10968=ORIENTED_EDGE('',*,*,#8327,.T.);
#10969=ORIENTED_EDGE('',*,*,#8362,.T.);
#10970=ORIENTED_EDGE('',*,*,#8339,.T.);
#10971=ORIENTED_EDGE('',*,*,#8332,.T.);
#10972=ORIENTED_EDGE('',*,*,#8370,.T.);
#10973=ORIENTED_EDGE('',*,*,#8330,.T.);
#10974=ORIENTED_EDGE('',*,*,#8338,.T.);
#10975=ORIENTED_EDGE('',*,*,#8363,.T.);
#10976=ORIENTED_EDGE('',*,*,#8325,.F.);
#10977=ORIENTED_EDGE('',*,*,#8369,.T.);
#10978=ORIENTED_EDGE('',*,*,#8323,.T.);
#10979=ORIENTED_EDGE('',*,*,#8358,.T.);
#10980=ORIENTED_EDGE('',*,*,#8336,.T.);
#10981=ORIENTED_EDGE('',*,*,#8328,.T.);
#10982=ORIENTED_EDGE('',*,*,#8373,.T.);
#10983=ORIENTED_EDGE('',*,*,#8374,.T.);
#10984=ORIENTED_EDGE('',*,*,#8376,.T.);
#10985=ORIENTED_EDGE('',*,*,#8359,.T.);
#10986=ORIENTED_EDGE('',*,*,#8321,.F.);
#10987=ORIENTED_EDGE('',*,*,#8377,.F.);
#10988=ORIENTED_EDGE('',*,*,#8378,.T.);
#10989=ORIENTED_EDGE('',*,*,#8379,.T.);
#10990=ORIENTED_EDGE('',*,*,#8378,.F.);
#10991=ORIENTED_EDGE('',*,*,#8380,.F.);
#10992=ORIENTED_EDGE('',*,*,#8381,.F.);
#10993=ORIENTED_EDGE('',*,*,#8382,.F.);
#10994=ORIENTED_EDGE('',*,*,#8383,.F.);
#10995=ORIENTED_EDGE('',*,*,#8384,.F.);
#10996=ORIENTED_EDGE('',*,*,#8385,.F.);
#10997=ORIENTED_EDGE('',*,*,#8377,.T.);
#10998=ORIENTED_EDGE('',*,*,#8386,.T.);
#10999=ORIENTED_EDGE('',*,*,#8387,.T.);
#11000=ORIENTED_EDGE('',*,*,#8388,.T.);
#11001=ORIENTED_EDGE('',*,*,#8389,.T.);
#11002=ORIENTED_EDGE('',*,*,#8390,.T.);
#11003=ORIENTED_EDGE('',*,*,#8391,.T.);
#11004=ORIENTED_EDGE('',*,*,#8379,.F.);
#11005=ORIENTED_EDGE('',*,*,#8386,.F.);
#11006=ORIENTED_EDGE('',*,*,#8392,.F.);
#11007=ORIENTED_EDGE('',*,*,#8380,.T.);
#11008=ORIENTED_EDGE('',*,*,#8393,.T.);
#11009=ORIENTED_EDGE('',*,*,#8387,.F.);
#11010=ORIENTED_EDGE('',*,*,#8393,.F.);
#11011=ORIENTED_EDGE('',*,*,#8385,.T.);
#11012=ORIENTED_EDGE('',*,*,#8394,.T.);
#11013=ORIENTED_EDGE('',*,*,#8388,.F.);
#11014=ORIENTED_EDGE('',*,*,#8394,.F.);
#11015=ORIENTED_EDGE('',*,*,#8384,.T.);
#11016=ORIENTED_EDGE('',*,*,#8395,.T.);
#11017=ORIENTED_EDGE('',*,*,#8389,.F.);
#11018=ORIENTED_EDGE('',*,*,#8395,.F.);
#11019=ORIENTED_EDGE('',*,*,#8383,.T.);
#11020=ORIENTED_EDGE('',*,*,#8396,.T.);
#11021=ORIENTED_EDGE('',*,*,#8390,.F.);
#11022=ORIENTED_EDGE('',*,*,#8396,.F.);
#11023=ORIENTED_EDGE('',*,*,#8382,.T.);
#11024=ORIENTED_EDGE('',*,*,#8397,.T.);
#11025=ORIENTED_EDGE('',*,*,#8391,.F.);
#11026=ORIENTED_EDGE('',*,*,#8397,.F.);
#11027=ORIENTED_EDGE('',*,*,#8381,.T.);
#11028=ORIENTED_EDGE('',*,*,#8392,.T.);
#11029=ORIENTED_EDGE('',*,*,#8398,.T.);
#11030=ORIENTED_EDGE('',*,*,#8399,.T.);
#11031=ORIENTED_EDGE('',*,*,#8400,.F.);
#11032=ORIENTED_EDGE('',*,*,#8399,.F.);
#11033=ORIENTED_EDGE('',*,*,#8401,.T.);
#11034=ORIENTED_EDGE('',*,*,#8402,.T.);
#11035=ORIENTED_EDGE('',*,*,#8403,.T.);
#11036=ORIENTED_EDGE('',*,*,#8404,.T.);
#11037=ORIENTED_EDGE('',*,*,#8405,.T.);
#11038=ORIENTED_EDGE('',*,*,#8406,.T.);
#11039=ORIENTED_EDGE('',*,*,#8398,.F.);
#11040=ORIENTED_EDGE('',*,*,#8407,.F.);
#11041=ORIENTED_EDGE('',*,*,#8408,.F.);
#11042=ORIENTED_EDGE('',*,*,#8409,.F.);
#11043=ORIENTED_EDGE('',*,*,#8410,.F.);
#11044=ORIENTED_EDGE('',*,*,#8411,.F.);
#11045=ORIENTED_EDGE('',*,*,#8412,.F.);
#11046=ORIENTED_EDGE('',*,*,#8400,.T.);
#11047=ORIENTED_EDGE('',*,*,#8407,.T.);
#11048=ORIENTED_EDGE('',*,*,#8413,.F.);
#11049=ORIENTED_EDGE('',*,*,#8401,.F.);
#11050=ORIENTED_EDGE('',*,*,#8414,.T.);
#11051=ORIENTED_EDGE('',*,*,#8412,.T.);
#11052=ORIENTED_EDGE('',*,*,#8415,.F.);
#11053=ORIENTED_EDGE('',*,*,#8402,.F.);
#11054=ORIENTED_EDGE('',*,*,#8413,.T.);
#11055=ORIENTED_EDGE('',*,*,#8411,.T.);
#11056=ORIENTED_EDGE('',*,*,#8416,.F.);
#11057=ORIENTED_EDGE('',*,*,#8403,.F.);
#11058=ORIENTED_EDGE('',*,*,#8415,.T.);
#11059=ORIENTED_EDGE('',*,*,#8410,.T.);
#11060=ORIENTED_EDGE('',*,*,#8417,.F.);
#11061=ORIENTED_EDGE('',*,*,#8404,.F.);
#11062=ORIENTED_EDGE('',*,*,#8416,.T.);
#11063=ORIENTED_EDGE('',*,*,#8409,.T.);
#11064=ORIENTED_EDGE('',*,*,#8418,.F.);
#11065=ORIENTED_EDGE('',*,*,#8405,.F.);
#11066=ORIENTED_EDGE('',*,*,#8417,.T.);
#11067=ORIENTED_EDGE('',*,*,#8408,.T.);
#11068=ORIENTED_EDGE('',*,*,#8414,.F.);
#11069=ORIENTED_EDGE('',*,*,#8406,.F.);
#11070=ORIENTED_EDGE('',*,*,#8418,.T.);
#14121=PLANE('',#16042);
#14122=PLANE('',#16046);
#14123=PLANE('',#16050);
#14124=PLANE('',#16051);
#14125=PLANE('',#16052);
#14126=PLANE('',#16054);
#14127=PLANE('',#16056);
#14128=PLANE('',#16058);
#14129=PLANE('',#16059);
#14130=PLANE('',#16063);
#14131=PLANE('',#16067);
#14132=PLANE('',#16068);
#14133=PLANE('',#16069);
#14134=PLANE('',#16071);
#14135=PLANE('',#16073);
#14136=PLANE('',#16075);
#14137=PLANE('',#16076);
#14138=PLANE('',#16080);
#14139=PLANE('',#16084);
#14140=PLANE('',#16085);
#14141=PLANE('',#16086);
#14142=PLANE('',#16088);
#14143=PLANE('',#16090);
#14144=PLANE('',#16092);
#14145=PLANE('',#16102);
#14146=PLANE('',#16103);
#14147=PLANE('',#16104);
#14148=PLANE('',#16105);
#14149=PLANE('',#16106);
#14150=PLANE('',#16107);
#14151=PLANE('',#16111);
#14152=PLANE('',#16113);
#14153=PLANE('',#16115);
#14154=PLANE('',#16116);
#14155=PLANE('',#16117);
#14156=PLANE('',#16119);
#14157=PLANE('',#16120);
#14158=PLANE('',#16130);
#14159=PLANE('',#16131);
#14160=PLANE('',#16132);
#14161=PLANE('',#16133);
#14162=PLANE('',#16134);
#14163=PLANE('',#16135);
#14164=PLANE('',#16139);
#14165=PLANE('',#16141);
#14166=PLANE('',#16143);
#14167=PLANE('',#16144);
#14168=PLANE('',#16145);
#14169=PLANE('',#16147);
#14170=PLANE('',#16148);
#14171=PLANE('',#16161);
#14172=PLANE('',#16162);
#14173=PLANE('',#16163);
#14174=PLANE('',#16167);
#14175=PLANE('',#16170);
#14176=PLANE('',#16171);
#14177=PLANE('',#16172);
#14178=PLANE('',#16174);
#14179=PLANE('',#16176);
#14180=PLANE('',#16179);
#14181=PLANE('',#16180);
#14182=PLANE('',#16181);
#14183=PLANE('',#16182);
#14184=PLANE('',#16183);
#14185=PLANE('',#16187);
#14186=PLANE('',#16189);
#14187=PLANE('',#16191);
#14188=PLANE('',#16192);
#14189=PLANE('',#16193);
#14190=PLANE('',#16195);
#14191=PLANE('',#16196);
#14192=PLANE('',#16200);
#14193=PLANE('',#16202);
#14194=PLANE('',#16204);
#14195=PLANE('',#16205);
#14196=PLANE('',#16206);
#14197=PLANE('',#16208);
#14198=PLANE('',#16209);
#14778=ADVANCED_FACE('',(#1810),#14121,.T.);
#14779=ADVANCED_FACE('',(#1811),#14122,.T.);
#14780=ADVANCED_FACE('',(#1812),#14123,.T.);
#14781=ADVANCED_FACE('',(#1813),#14124,.T.);
#14782=ADVANCED_FACE('',(#1814),#14125,.T.);
#14783=ADVANCED_FACE('',(#1815),#1141,.T.);
#14784=ADVANCED_FACE('',(#1816),#14126,.T.);
#14785=ADVANCED_FACE('',(#1817),#1142,.F.);
#14786=ADVANCED_FACE('',(#1818),#14127,.T.);
#14787=ADVANCED_FACE('',(#1819),#1143,.T.);
#14788=ADVANCED_FACE('',(#1820),#14128,.T.);
#14789=ADVANCED_FACE('',(#1821),#14129,.T.);
#14790=ADVANCED_FACE('',(#1822),#14130,.T.);
#14791=ADVANCED_FACE('',(#1823),#14131,.T.);
#14792=ADVANCED_FACE('',(#1824),#14132,.T.);
#14793=ADVANCED_FACE('',(#1825),#14133,.T.);
#14794=ADVANCED_FACE('',(#1826),#1144,.T.);
#14795=ADVANCED_FACE('',(#1827),#14134,.T.);
#14796=ADVANCED_FACE('',(#1828),#1145,.F.);
#14797=ADVANCED_FACE('',(#1829),#14135,.T.);
#14798=ADVANCED_FACE('',(#1830),#1146,.T.);
#14799=ADVANCED_FACE('',(#1831),#14136,.T.);
#14800=ADVANCED_FACE('',(#1832),#14137,.T.);
#14801=ADVANCED_FACE('',(#1833),#14138,.T.);
#14802=ADVANCED_FACE('',(#1834),#14139,.T.);
#14803=ADVANCED_FACE('',(#1835),#14140,.T.);
#14804=ADVANCED_FACE('',(#1836),#14141,.T.);
#14805=ADVANCED_FACE('',(#1837),#1147,.T.);
#14806=ADVANCED_FACE('',(#1838),#14142,.T.);
#14807=ADVANCED_FACE('',(#1839),#1148,.F.);
#14808=ADVANCED_FACE('',(#1840),#14143,.T.);
#14809=ADVANCED_FACE('',(#1841),#1149,.T.);
#14810=ADVANCED_FACE('',(#1842),#14144,.T.);
#14811=ADVANCED_FACE('',(#1843),#1150,.F.);
#14812=ADVANCED_FACE('',(#1844),#1151,.T.);
#14813=ADVANCED_FACE('',(#1845),#1152,.F.);
#14814=ADVANCED_FACE('',(#1846),#14145,.T.);
#14815=ADVANCED_FACE('',(#1847),#14146,.T.);
#14816=ADVANCED_FACE('',(#1848),#14147,.T.);
#14817=ADVANCED_FACE('',(#1849),#14148,.T.);
#14818=ADVANCED_FACE('',(#1850,#1579),#14149,.F.);
#14819=ADVANCED_FACE('',(#1851,#1580),#14150,.T.);
#14820=ADVANCED_FACE('',(#1852),#1153,.F.);
#14821=ADVANCED_FACE('',(#1853,#1581),#14151,.F.);
#14822=ADVANCED_FACE('',(#1854,#1582),#14152,.T.);
#14823=ADVANCED_FACE('',(#1855),#14153,.F.);
#14824=ADVANCED_FACE('',(#1856),#14154,.F.);
#14825=ADVANCED_FACE('',(#1857),#14155,.F.);
#14826=ADVANCED_FACE('',(#1858),#1154,.T.);
#14827=ADVANCED_FACE('',(#1859),#14156,.F.);
#14828=ADVANCED_FACE('',(#1860),#14157,.F.);
#14829=ADVANCED_FACE('',(#1861),#1155,.F.);
#14830=ADVANCED_FACE('',(#1862),#1156,.T.);
#14831=ADVANCED_FACE('',(#1863),#1157,.F.);
#14832=ADVANCED_FACE('',(#1864),#14158,.T.);
#14833=ADVANCED_FACE('',(#1865),#14159,.T.);
#14834=ADVANCED_FACE('',(#1866),#14160,.T.);
#14835=ADVANCED_FACE('',(#1867),#14161,.T.);
#14836=ADVANCED_FACE('',(#1868,#1583),#14162,.F.);
#14837=ADVANCED_FACE('',(#1869,#1584),#14163,.T.);
#14838=ADVANCED_FACE('',(#1870),#1158,.F.);
#14839=ADVANCED_FACE('',(#1871,#1585),#14164,.F.);
#14840=ADVANCED_FACE('',(#1872,#1586),#14165,.T.);
#14841=ADVANCED_FACE('',(#1873),#14166,.F.);
#14842=ADVANCED_FACE('',(#1874),#14167,.F.);
#14843=ADVANCED_FACE('',(#1875),#14168,.F.);
#14844=ADVANCED_FACE('',(#1876),#1159,.T.);
#14845=ADVANCED_FACE('',(#1877),#14169,.F.);
#14846=ADVANCED_FACE('',(#1878),#14170,.F.);
#14847=ADVANCED_FACE('',(#1879),#1160,.F.);
#14848=ADVANCED_FACE('',(#1880),#1161,.F.);
#14849=ADVANCED_FACE('',(#1881),#1162,.T.);
#14850=ADVANCED_FACE('',(#1882),#1163,.T.);
#14851=ADVANCED_FACE('',(#1883),#14171,.T.);
#14852=ADVANCED_FACE('',(#1884),#14172,.T.);
#14853=ADVANCED_FACE('',(#1885),#14173,.T.);
#14854=ADVANCED_FACE('',(#1886),#14174,.T.);
#14855=ADVANCED_FACE('',(#1887),#14175,.T.);
#14856=ADVANCED_FACE('',(#1888),#14176,.T.);
#14857=ADVANCED_FACE('',(#1889),#14177,.T.);
#14858=ADVANCED_FACE('',(#1890),#1164,.T.);
#14859=ADVANCED_FACE('',(#1891),#14178,.T.);
#14860=ADVANCED_FACE('',(#1892),#1165,.F.);
#14861=ADVANCED_FACE('',(#1893),#14179,.T.);
#14862=ADVANCED_FACE('',(#1894),#1166,.T.);
#14863=ADVANCED_FACE('',(#1895),#14180,.T.);
#14864=ADVANCED_FACE('',(#1896),#14181,.F.);
#14865=ADVANCED_FACE('',(#1897),#14182,.F.);
#14866=ADVANCED_FACE('',(#1898),#14183,.F.);
#14867=ADVANCED_FACE('',(#1899),#14184,.F.);
#14868=ADVANCED_FACE('',(#1900),#1167,.F.);
#14869=ADVANCED_FACE('',(#1901,#1587),#14185,.F.);
#14870=ADVANCED_FACE('',(#1902,#1588),#14186,.T.);
#14871=ADVANCED_FACE('',(#1903),#14187,.F.);
#14872=ADVANCED_FACE('',(#1904),#14188,.F.);
#14873=ADVANCED_FACE('',(#1905),#14189,.F.);
#14874=ADVANCED_FACE('',(#1906),#1168,.T.);
#14875=ADVANCED_FACE('',(#1907),#14190,.F.);
#14876=ADVANCED_FACE('',(#1908),#14191,.F.);
#14877=ADVANCED_FACE('',(#1909),#1169,.F.);
#14878=ADVANCED_FACE('',(#1910,#1589),#14192,.F.);
#14879=ADVANCED_FACE('',(#1911,#1590),#14193,.T.);
#14880=ADVANCED_FACE('',(#1912),#14194,.F.);
#14881=ADVANCED_FACE('',(#1913),#14195,.F.);
#14882=ADVANCED_FACE('',(#1914),#14196,.F.);
#14883=ADVANCED_FACE('',(#1915),#1170,.T.);
#14884=ADVANCED_FACE('',(#1916),#14197,.F.);
#14885=ADVANCED_FACE('',(#1917),#14198,.F.);
#15553=CLOSED_SHELL('',(#14778,#14779,#14780,#14781,#14782,#14783,#14784,
#14785,#14786,#14787,#14788));
#15554=CLOSED_SHELL('',(#14789,#14790,#14791,#14792,#14793,#14794,#14795,
#14796,#14797,#14798,#14799));
#15555=CLOSED_SHELL('',(#14800,#14801,#14802,#14803,#14804,#14805,#14806,
#14807,#14808,#14809,#14810));
#15556=CLOSED_SHELL('',(#14811,#14812,#14813,#14814,#14815,#14816,#14817,
#14818,#14819));
#15557=CLOSED_SHELL('',(#14820,#14821,#14822,#14823,#14824,#14825,#14826,
#14827,#14828));
#15558=CLOSED_SHELL('',(#14829,#14830,#14831,#14832,#14833,#14834,#14835,
#14836,#14837));
#15559=CLOSED_SHELL('',(#14838,#14839,#14840,#14841,#14842,#14843,#14844,
#14845,#14846));
#15560=CLOSED_SHELL('',(#14847,#14848,#14849,#14850,#14851,#14852,#14853,
#14854,#14855,#14856,#14857,#14858,#14859,#14860,#14861,#14862,#14863,#14864,
#14865,#14866,#14867));
#15561=CLOSED_SHELL('',(#14868,#14869,#14870,#14871,#14872,#14873,#14874,
#14875,#14876));
#15562=CLOSED_SHELL('',(#14877,#14878,#14879,#14880,#14881,#14882,#14883,
#14884,#14885));
#16041=AXIS2_PLACEMENT_3D('',#21977,#17871,#17872);
#16042=AXIS2_PLACEMENT_3D('',#21978,#17873,#17874);
#16043=AXIS2_PLACEMENT_3D('',#21989,#17879,#17880);
#16044=AXIS2_PLACEMENT_3D('',#21993,#17882,#17883);
#16045=AXIS2_PLACEMENT_3D('',#21996,#17885,#17886);
#16046=AXIS2_PLACEMENT_3D('',#21997,#17887,#17888);
#16047=AXIS2_PLACEMENT_3D('',#22004,#17891,#17892);
#16048=AXIS2_PLACEMENT_3D('',#22008,#17894,#17895);
#16049=AXIS2_PLACEMENT_3D('',#22012,#17897,#17898);
#16050=AXIS2_PLACEMENT_3D('',#22016,#17901,#17902);
#16051=AXIS2_PLACEMENT_3D('',#22019,#17905,#17906);
#16052=AXIS2_PLACEMENT_3D('',#22021,#17908,#17909);
#16053=AXIS2_PLACEMENT_3D('',#22023,#17911,#17912);
#16054=AXIS2_PLACEMENT_3D('',#22025,#17914,#17915);
#16055=AXIS2_PLACEMENT_3D('',#22027,#17917,#17918);
#16056=AXIS2_PLACEMENT_3D('',#22029,#17920,#17921);
#16057=AXIS2_PLACEMENT_3D('',#22031,#17923,#17924);
#16058=AXIS2_PLACEMENT_3D('',#22033,#17926,#17927);
#16059=AXIS2_PLACEMENT_3D('',#22034,#17928,#17929);
#16060=AXIS2_PLACEMENT_3D('',#22039,#17931,#17932);
#16061=AXIS2_PLACEMENT_3D('',#22043,#17934,#17935);
#16062=AXIS2_PLACEMENT_3D('',#22047,#17937,#17938);
#16063=AXIS2_PLACEMENT_3D('',#22053,#17942,#17943);
#16064=AXIS2_PLACEMENT_3D('',#22062,#17947,#17948);
#16065=AXIS2_PLACEMENT_3D('',#22066,#17950,#17951);
#16066=AXIS2_PLACEMENT_3D('',#22070,#17953,#17954);
#16067=AXIS2_PLACEMENT_3D('',#22072,#17956,#17957);
#16068=AXIS2_PLACEMENT_3D('',#22075,#17960,#17961);
#16069=AXIS2_PLACEMENT_3D('',#22077,#17963,#17964);
#16070=AXIS2_PLACEMENT_3D('',#22079,#17966,#17967);
#16071=AXIS2_PLACEMENT_3D('',#22081,#17969,#17970);
#16072=AXIS2_PLACEMENT_3D('',#22083,#17972,#17973);
#16073=AXIS2_PLACEMENT_3D('',#22085,#17975,#17976);
#16074=AXIS2_PLACEMENT_3D('',#22087,#17978,#17979);
#16075=AXIS2_PLACEMENT_3D('',#22089,#17981,#17982);
#16076=AXIS2_PLACEMENT_3D('',#22090,#17983,#17984);
#16077=AXIS2_PLACEMENT_3D('',#22095,#17986,#17987);
#16078=AXIS2_PLACEMENT_3D('',#22099,#17989,#17990);
#16079=AXIS2_PLACEMENT_3D('',#22103,#17992,#17993);
#16080=AXIS2_PLACEMENT_3D('',#22109,#17997,#17998);
#16081=AXIS2_PLACEMENT_3D('',#22118,#18002,#18003);
#16082=AXIS2_PLACEMENT_3D('',#22122,#18005,#18006);
#16083=AXIS2_PLACEMENT_3D('',#22126,#18008,#18009);
#16084=AXIS2_PLACEMENT_3D('',#22128,#18011,#18012);
#16085=AXIS2_PLACEMENT_3D('',#22131,#18015,#18016);
#16086=AXIS2_PLACEMENT_3D('',#22133,#18018,#18019);
#16087=AXIS2_PLACEMENT_3D('',#22135,#18021,#18022);
#16088=AXIS2_PLACEMENT_3D('',#22137,#18024,#18025);
#16089=AXIS2_PLACEMENT_3D('',#22139,#18027,#18028);
#16090=AXIS2_PLACEMENT_3D('',#22141,#18030,#18031);
#16091=AXIS2_PLACEMENT_3D('',#22143,#18033,#18034);
#16092=AXIS2_PLACEMENT_3D('',#22145,#18036,#18037);
#16093=AXIS2_PLACEMENT_3D('',#22146,#18038,#18039);
#16094=AXIS2_PLACEMENT_3D('',#22148,#18040,#18041);
#16095=AXIS2_PLACEMENT_3D('',#22151,#18043,#18044);
#16096=AXIS2_PLACEMENT_3D('',#22152,#18045,#18046);
#16097=AXIS2_PLACEMENT_3D('',#22155,#18047,#18048);
#16098=AXIS2_PLACEMENT_3D('',#22159,#18050,#18051);
#16099=AXIS2_PLACEMENT_3D('',#22161,#18053,#18054);
#16100=AXIS2_PLACEMENT_3D('',#22163,#18055,#18056);
#16101=AXIS2_PLACEMENT_3D('',#22166,#18058,#18059);
#16102=AXIS2_PLACEMENT_3D('',#22167,#18060,#18061);
#16103=AXIS2_PLACEMENT_3D('',#22173,#18065,#18066);
#16104=AXIS2_PLACEMENT_3D('',#22179,#18070,#18071);
#16105=AXIS2_PLACEMENT_3D('',#22185,#18075,#18076);
#16106=AXIS2_PLACEMENT_3D('',#22188,#18079,#18080);
#16107=AXIS2_PLACEMENT_3D('',#22189,#18081,#18082);
#16108=AXIS2_PLACEMENT_3D('',#22190,#18083,#18084);
#16109=AXIS2_PLACEMENT_3D('',#22192,#18085,#18086);
#16110=AXIS2_PLACEMENT_3D('',#22195,#18088,#18089);
#16111=AXIS2_PLACEMENT_3D('',#22196,#18090,#18091);
#16112=AXIS2_PLACEMENT_3D('',#22205,#18095,#18096);
#16113=AXIS2_PLACEMENT_3D('',#22209,#18099,#18100);
#16114=AXIS2_PLACEMENT_3D('',#22218,#18104,#18105);
#16115=AXIS2_PLACEMENT_3D('',#22222,#18108,#18109);
#16116=AXIS2_PLACEMENT_3D('',#22225,#18112,#18113);
#16117=AXIS2_PLACEMENT_3D('',#22227,#18115,#18116);
#16118=AXIS2_PLACEMENT_3D('',#22229,#18118,#18119);
#16119=AXIS2_PLACEMENT_3D('',#22231,#18121,#18122);
#16120=AXIS2_PLACEMENT_3D('',#22233,#18124,#18125);
#16121=AXIS2_PLACEMENT_3D('',#22234,#18126,#18127);
#16122=AXIS2_PLACEMENT_3D('',#22236,#18128,#18129);
#16123=AXIS2_PLACEMENT_3D('',#22239,#18131,#18132);
#16124=AXIS2_PLACEMENT_3D('',#22240,#18133,#18134);
#16125=AXIS2_PLACEMENT_3D('',#22243,#18135,#18136);
#16126=AXIS2_PLACEMENT_3D('',#22247,#18138,#18139);
#16127=AXIS2_PLACEMENT_3D('',#22249,#18141,#18142);
#16128=AXIS2_PLACEMENT_3D('',#22251,#18143,#18144);
#16129=AXIS2_PLACEMENT_3D('',#22253,#18145,#18146);
#16130=AXIS2_PLACEMENT_3D('',#22255,#18148,#18149);
#16131=AXIS2_PLACEMENT_3D('',#22261,#18153,#18154);
#16132=AXIS2_PLACEMENT_3D('',#22267,#18158,#18159);
#16133=AXIS2_PLACEMENT_3D('',#22273,#18163,#18164);
#16134=AXIS2_PLACEMENT_3D('',#22276,#18167,#18168);
#16135=AXIS2_PLACEMENT_3D('',#22277,#18169,#18170);
#16136=AXIS2_PLACEMENT_3D('',#22278,#18171,#18172);
#16137=AXIS2_PLACEMENT_3D('',#22280,#18173,#18174);
#16138=AXIS2_PLACEMENT_3D('',#22283,#18176,#18177);
#16139=AXIS2_PLACEMENT_3D('',#22284,#18178,#18179);
#16140=AXIS2_PLACEMENT_3D('',#22293,#18183,#18184);
#16141=AXIS2_PLACEMENT_3D('',#22297,#18187,#18188);
#16142=AXIS2_PLACEMENT_3D('',#22306,#18192,#18193);
#16143=AXIS2_PLACEMENT_3D('',#22310,#18196,#18197);
#16144=AXIS2_PLACEMENT_3D('',#22313,#18200,#18201);
#16145=AXIS2_PLACEMENT_3D('',#22315,#18203,#18204);
#16146=AXIS2_PLACEMENT_3D('',#22317,#18206,#18207);
#16147=AXIS2_PLACEMENT_3D('',#22319,#18209,#18210);
#16148=AXIS2_PLACEMENT_3D('',#22321,#18212,#18213);
#16149=AXIS2_PLACEMENT_3D('',#22322,#18214,#18215);
#16150=AXIS2_PLACEMENT_3D('',#22325,#18216,#18217);
#16151=AXIS2_PLACEMENT_3D('',#22329,#18219,#18220);
#16152=AXIS2_PLACEMENT_3D('',#22331,#18222,#18223);
#16153=AXIS2_PLACEMENT_3D('',#22334,#18224,#18225);
#16154=AXIS2_PLACEMENT_3D('',#22338,#18227,#18228);
#16155=AXIS2_PLACEMENT_3D('',#22340,#18230,#18231);
#16156=AXIS2_PLACEMENT_3D('',#22343,#18232,#18233);
#16157=AXIS2_PLACEMENT_3D('',#22347,#18235,#18236);
#16158=AXIS2_PLACEMENT_3D('',#22349,#18238,#18239);
#16159=AXIS2_PLACEMENT_3D('',#22352,#18240,#18241);
#16160=AXIS2_PLACEMENT_3D('',#22356,#18243,#18244);
#16161=AXIS2_PLACEMENT_3D('',#22358,#18246,#18247);
#16162=AXIS2_PLACEMENT_3D('',#22364,#18251,#18252);
#16163=AXIS2_PLACEMENT_3D('',#22370,#18256,#18257);
#16164=AXIS2_PLACEMENT_3D('',#22375,#18259,#18260);
#16165=AXIS2_PLACEMENT_3D('',#22379,#18262,#18263);
#16166=AXIS2_PLACEMENT_3D('',#22383,#18265,#18266);
#16167=AXIS2_PLACEMENT_3D('',#22389,#18270,#18271);
#16168=AXIS2_PLACEMENT_3D('',#22397,#18275,#18276);
#16169=AXIS2_PLACEMENT_3D('',#22401,#18278,#18279);
#16170=AXIS2_PLACEMENT_3D('',#22403,#18281,#18282);
#16171=AXIS2_PLACEMENT_3D('',#22411,#18289,#18290);
#16172=AXIS2_PLACEMENT_3D('',#22413,#18292,#18293);
#16173=AXIS2_PLACEMENT_3D('',#22415,#18295,#18296);
#16174=AXIS2_PLACEMENT_3D('',#22417,#18298,#18299);
#16175=AXIS2_PLACEMENT_3D('',#22419,#18301,#18302);
#16176=AXIS2_PLACEMENT_3D('',#22421,#18304,#18305);
#16177=AXIS2_PLACEMENT_3D('',#22428,#18311,#18312);
#16178=AXIS2_PLACEMENT_3D('',#22430,#18313,#18314);
#16179=AXIS2_PLACEMENT_3D('',#22432,#18316,#18317);
#16180=AXIS2_PLACEMENT_3D('',#22434,#18319,#18320);
#16181=AXIS2_PLACEMENT_3D('',#22435,#18321,#18322);
#16182=AXIS2_PLACEMENT_3D('',#22436,#18323,#18324);
#16183=AXIS2_PLACEMENT_3D('',#22437,#18325,#18326);
#16184=AXIS2_PLACEMENT_3D('',#22438,#18327,#18328);
#16185=AXIS2_PLACEMENT_3D('',#22440,#18329,#18330);
#16186=AXIS2_PLACEMENT_3D('',#22443,#18332,#18333);
#16187=AXIS2_PLACEMENT_3D('',#22444,#18334,#18335);
#16188=AXIS2_PLACEMENT_3D('',#22453,#18339,#18340);
#16189=AXIS2_PLACEMENT_3D('',#22457,#18343,#18344);
#16190=AXIS2_PLACEMENT_3D('',#22466,#18348,#18349);
#16191=AXIS2_PLACEMENT_3D('',#22470,#18352,#18353);
#16192=AXIS2_PLACEMENT_3D('',#22473,#18356,#18357);
#16193=AXIS2_PLACEMENT_3D('',#22475,#18359,#18360);
#16194=AXIS2_PLACEMENT_3D('',#22477,#18362,#18363);
#16195=AXIS2_PLACEMENT_3D('',#22479,#18365,#18366);
#16196=AXIS2_PLACEMENT_3D('',#22481,#18368,#18369);
#16197=AXIS2_PLACEMENT_3D('',#22482,#18370,#18371);
#16198=AXIS2_PLACEMENT_3D('',#22484,#18372,#18373);
#16199=AXIS2_PLACEMENT_3D('',#22487,#18375,#18376);
#16200=AXIS2_PLACEMENT_3D('',#22488,#18377,#18378);
#16201=AXIS2_PLACEMENT_3D('',#22497,#18382,#18383);
#16202=AXIS2_PLACEMENT_3D('',#22501,#18386,#18387);
#16203=AXIS2_PLACEMENT_3D('',#22510,#18391,#18392);
#16204=AXIS2_PLACEMENT_3D('',#22514,#18395,#18396);
#16205=AXIS2_PLACEMENT_3D('',#22517,#18399,#18400);
#16206=AXIS2_PLACEMENT_3D('',#22519,#18402,#18403);
#16207=AXIS2_PLACEMENT_3D('',#22521,#18405,#18406);
#16208=AXIS2_PLACEMENT_3D('',#22523,#18408,#18409);
#16209=AXIS2_PLACEMENT_3D('',#22525,#18411,#18412);
#17871=DIRECTION('axis',(0.,0.,1.));
#17872=DIRECTION('refdir',(1.,0.,0.));
#17873=DIRECTION('center_axis',(0.707106781186548,-9.87540052432906E-15,
-0.707106781186548));
#17874=DIRECTION('ref_axis',(-0.707106781186548,-7.45999389735652E-32,-0.707106781186548));
#17875=DIRECTION('',(-6.98296267768627E-15,-1.,6.98296267768627E-15));
#17876=DIRECTION('',(-0.707106781186547,-5.66993775627602E-31,-0.707106781186547));
#17877=DIRECTION('',(-4.37653262704222E-17,1.,-1.4009690681643E-14));
#17878=DIRECTION('',(0.707106781186547,-4.93770026216453E-15,0.707106781186547));
#17879=DIRECTION('center_axis',(-0.707106781186503,5.10171234491475E-14,
0.707106781186592));
#17880=DIRECTION('ref_axis',(0.707106781186592,4.06006286315216E-13,0.707106781186503));
#17881=DIRECTION('',(2.82341939598128E-17,-1.,1.39941595493323E-14));
#17882=DIRECTION('center_axis',(0.707106781186548,-8.6849455722553E-15,
-0.707106781186547));
#17883=DIRECTION('ref_axis',(0.707106781186547,1.24067126081198E-13,0.707106781186548));
#17884=DIRECTION('',(0.707106781186547,-1.10208153157725E-17,0.707106781186547));
#17885=DIRECTION('center_axis',(-0.707106781186547,1.44247999773054E-14,
0.707106781186548));
#17886=DIRECTION('ref_axis',(0.707106781186548,2.09065760029798E-13,0.707106781186547));
#17887=DIRECTION('center_axis',(0.707106781186548,9.87540052432906E-15,
0.707106781186547));
#17888=DIRECTION('ref_axis',(0.707106781186547,-7.45999389735652E-32,-0.707106781186548));
#17889=DIRECTION('',(0.707106781186548,5.66993775627602E-31,-0.707106781186548));
#17890=DIRECTION('',(6.98296267768627E-15,1.,-2.09488880330588E-14));
#17891=DIRECTION('center_axis',(-0.70710678118655,-2.33342352574054E-15,
-0.707106781186545));
#17892=DIRECTION('ref_axis',(0.707106781186545,-3.39200069252924E-13,-0.70710678118655));
#17893=DIRECTION('',(-0.707106781186548,1.10208153157725E-17,0.707106781186548));
#17894=DIRECTION('center_axis',(0.707106781186561,3.37058601970852E-14,
0.707106781186534));
#17895=DIRECTION('ref_axis',(0.707106781186534,2.01365616121726E-13,-0.707106781186561));
#17896=DIRECTION('',(-2.82341939598121E-17,1.,-1.39376911614127E-14));
#17897=DIRECTION('center_axis',(-0.707106781186548,-1.42126705658744E-14,
-0.707106781186547));
#17898=DIRECTION('ref_axis',(0.707106781186547,-3.72911172953344E-14,-0.707106781186548));
#17899=DIRECTION('',(-0.707106781186548,4.93770026216453E-15,0.707106781186548));
#17900=DIRECTION('',(4.37653262704214E-17,-1.,1.39221600291021E-14));
#17901=DIRECTION('center_axis',(-7.88860896404804E-31,1.,2.05680528781315E-77));
#17902=DIRECTION('ref_axis',(-1.,-7.88860896404804E-31,-1.16649095722751E-39));
#17903=DIRECTION('',(1.16649072924818E-39,0.,1.));
#17904=DIRECTION('',(1.16649072924818E-39,0.,1.));
#17905=DIRECTION('center_axis',(1.,4.37653262704214E-17,-3.42470776094434E-41));
#17906=DIRECTION('ref_axis',(-4.37653262704214E-17,1.,-4.04863581862828E-74));
#17907=DIRECTION('',(1.16649072924818E-39,0.,1.));
#17908=DIRECTION('center_axis',(-6.98296267768627E-15,-1.,0.));
#17909=DIRECTION('ref_axis',(1.,-6.98296267768627E-15,1.76663133728356E-39));
#17910=DIRECTION('',(1.16649072924818E-39,0.,1.));
#17911=DIRECTION('center_axis',(1.16649072924818E-39,0.,1.));
#17912=DIRECTION('ref_axis',(1.,0.,-1.16649072924818E-39));
#17913=DIRECTION('',(1.16649072924818E-39,0.,1.));
#17914=DIRECTION('center_axis',(-1.,-2.82341939598121E-17,-1.14077343289525E-39));
#17915=DIRECTION('ref_axis',(2.82341939598121E-17,-1.,9.93228473184302E-73));
#17916=DIRECTION('',(1.16649072924818E-39,0.,1.));
#17917=DIRECTION('center_axis',(1.16649072924818E-39,0.,1.));
#17918=DIRECTION('ref_axis',(1.,0.,-1.16649072924818E-39));
#17919=DIRECTION('',(1.16649072924818E-39,0.,1.));
#17920=DIRECTION('center_axis',(-1.55857864879746E-17,-1.,0.));
#17921=DIRECTION('ref_axis',(1.,-1.55857864879746E-17,1.48465414644535E-38));
#17922=DIRECTION('',(1.16649072924818E-39,0.,1.));
#17923=DIRECTION('center_axis',(1.16649072924818E-39,0.,1.));
#17924=DIRECTION('ref_axis',(1.,0.,-1.16649072924818E-39));
#17925=DIRECTION('',(1.16649072924818E-39,0.,1.));
#17926=DIRECTION('center_axis',(-1.,6.98296267768627E-15,1.17210418944755E-39));
#17927=DIRECTION('ref_axis',(-6.98296267768627E-15,-1.,1.56236334624413E-70));
#17928=DIRECTION('center_axis',(-0.707106781186547,9.76996261670137E-15,
0.707106781186548));
#17929=DIRECTION('ref_axis',(0.707106781186548,-1.25110045007797E-31,0.707106781186547));
#17930=DIRECTION('',(2.09488879640879E-14,1.,6.93889390390723E-15));
#17931=DIRECTION('center_axis',(0.707106781186556,6.78814116579064E-15,
-0.707106781186539));
#17932=DIRECTION('ref_axis',(0.707106781186539,8.68490834600899E-15,0.707106781186556));
#17933=DIRECTION('',(-0.707106781186548,5.55111512312578E-17,-0.707106781186548));
#17934=DIRECTION('center_axis',(-0.707106781186566,-1.56122235882211E-14,
0.707106781186529));
#17935=DIRECTION('ref_axis',(0.707106781186529,7.38317989499037E-14,0.707106781186566));
#17936=DIRECTION('',(1.39376911160448E-14,1.,0.));
#17937=DIRECTION('center_axis',(0.707106781186543,-2.20614587888198E-14,
-0.707106781186552));
#17938=DIRECTION('ref_axis',(0.707106781186552,5.51055984241866E-14,0.707106781186543));
#17939=DIRECTION('',(-0.707106781186548,4.94049245958195E-15,-0.707106781186548));
#17940=DIRECTION('',(-1.39221599728635E-14,-1.,0.));
#17941=DIRECTION('',(0.707106781186548,0.,0.707106781186548));
#17942=DIRECTION('center_axis',(0.707106781186548,-4.94049245958195E-15,
0.707106781186548));
#17943=DIRECTION('ref_axis',(0.707106781186548,5.55111512312576E-17,-0.707106781186548));
#17944=DIRECTION('',(0.707106781186547,5.55111512312578E-17,-0.707106781186547));
#17945=DIRECTION('',(7.02672793828483E-15,1.,0.));
#17946=DIRECTION('',(-0.707106781186547,-4.99600361081321E-15,0.707106781186547));
#17947=DIRECTION('center_axis',(-0.707106781186547,8.69730586866938E-15,
-0.707106781186548));
#17948=DIRECTION('ref_axis',(0.707106781186548,1.59821939493797E-13,-0.707106781186547));
#17949=DIRECTION('',(-7.01119682157331E-15,-1.,0.));
#17950=DIRECTION('center_axis',(0.707106781186539,2.04716574203159E-14,
0.707106781186556));
#17951=DIRECTION('ref_axis',(0.707106781186556,4.33830102985163E-13,-0.707106781186539));
#17952=DIRECTION('',(-0.707106781186547,-5.55111512312578E-17,0.707106781186547));
#17953=DIRECTION('center_axis',(-0.707106781186547,8.69730586866915E-15,
-0.707106781186548));
#17954=DIRECTION('ref_axis',(0.707106781186548,-6.72197636050009E-14,-0.707106781186547));
#17955=DIRECTION('',(7.94093388050907E-23,-1.,-6.93889390390723E-15));
#17956=DIRECTION('center_axis',(-5.29395592033938E-23,1.,-1.40129846432482E-45));
#17957=DIRECTION('ref_axis',(-2.64697796016969E-23,0.,1.));
#17958=DIRECTION('',(-1.,5.29395592033937E-23,2.64697796016969E-23));
#17959=DIRECTION('',(-1.,5.29395592033937E-23,2.64697796016969E-23));
#17960=DIRECTION('center_axis',(-2.64697796016969E-23,-1.40129846432482E-45,
1.));
#17961=DIRECTION('ref_axis',(5.29395592033938E-23,-1.,0.));
#17962=DIRECTION('',(-1.,5.29395592033937E-23,2.64697796016969E-23));
#17963=DIRECTION('center_axis',(7.94093388050907E-23,-1.,-7.04991620636974E-15));
#17964=DIRECTION('ref_axis',(2.64697796016969E-23,7.04991620636974E-15,
-1.));
#17965=DIRECTION('',(-1.,5.29395592033937E-23,2.64697796016969E-23));
#17966=DIRECTION('center_axis',(-1.,5.29395592033937E-23,2.64697796016969E-23));
#17967=DIRECTION('ref_axis',(2.64697796016969E-23,-1.40129846432482E-45,
1.));
#17968=DIRECTION('',(-1.,5.29395592033937E-23,2.64697796016969E-23));
#17969=DIRECTION('center_axis',(2.64697796016969E-23,1.40129846432482E-45,
-1.));
#17970=DIRECTION('ref_axis',(-5.29395592033938E-23,1.,0.));
#17971=DIRECTION('',(-1.,5.29395592033937E-23,2.64697796016969E-23));
#17972=DIRECTION('center_axis',(-1.,5.29395592033937E-23,2.64697796016969E-23));
#17973=DIRECTION('ref_axis',(2.64697796016969E-23,-1.40129846432481E-45,
1.));
#17974=DIRECTION('',(-1.,5.29395592033937E-23,2.64697796016969E-23));
#17975=DIRECTION('center_axis',(5.29395592033938E-23,-1.,1.40129846432482E-45));
#17976=DIRECTION('ref_axis',(2.64697796016969E-23,0.,-1.));
#17977=DIRECTION('',(-1.,5.29395592033937E-23,2.64697796016969E-23));
#17978=DIRECTION('center_axis',(-1.,5.29395592033937E-23,2.64697796016969E-23));
#17979=DIRECTION('ref_axis',(2.64697796016969E-23,-1.40129846432482E-45,
1.));
#17980=DIRECTION('',(-1.,5.29395592033937E-23,2.64697796016969E-23));
#17981=DIRECTION('center_axis',(2.64697796016969E-23,6.93889390390723E-15,
-1.));
#17982=DIRECTION('ref_axis',(-7.94093388050907E-23,1.,6.93889390390723E-15));
#17983=DIRECTION('center_axis',(0.707106781186548,4.99600361081321E-15,
-0.707106781186548));
#17984=DIRECTION('ref_axis',(-0.707106781186548,5.55111512312577E-17,-0.707106781186548));
#17985=DIRECTION('',(-1.39659253976245E-14,1.,-7.105427357601E-15));
#17986=DIRECTION('center_axis',(-0.70710678118654,-1.56975764458909E-14,
0.707106781186555));
#17987=DIRECTION('ref_axis',(0.707106781186555,4.51903224902127E-13,0.70710678118654));
#17988=DIRECTION('',(0.707106781186547,-5.55111512312578E-17,0.707106781186547));
#17989=DIRECTION('center_axis',(0.707106781186556,-6.72049359757844E-15,
-0.707106781186539));
#17990=DIRECTION('ref_axis',(0.707106781186539,9.95355220102466E-14,0.707106781186556));
#17991=DIRECTION('',(-6.95472852311166E-15,1.,-1.66533453693773E-16));
#17992=DIRECTION('center_axis',(-0.707106781186548,-8.69730586866937E-15,
0.707106781186547));
#17993=DIRECTION('ref_axis',(0.707106781186547,7.11593649168016E-14,0.707106781186548));
#17994=DIRECTION('',(0.707106781186548,4.88498130835069E-15,0.707106781186548));
#17995=DIRECTION('',(6.93919737993036E-15,-1.,1.66533453693773E-16));
#17996=DIRECTION('',(-0.707106781186547,5.55111512312578E-17,-0.707106781186547));
#17997=DIRECTION('center_axis',(-0.707106781186548,-9.88098491916389E-15,
-0.707106781186547));
#17998=DIRECTION('ref_axis',(-0.707106781186547,-5.55111512312579E-17,0.707106781186548));
#17999=DIRECTION('',(-0.707106781186547,-5.55111512312578E-17,0.707106781186548));
#18000=DIRECTION('',(-1.40096907165064E-14,1.,-1.66533453693773E-16));
#18001=DIRECTION('',(0.707106781186547,-4.82947015711943E-15,-0.707106781186548));
#18002=DIRECTION('center_axis',(0.70710678118653,-2.81071470146027E-14,
0.707106781186565));
#18003=DIRECTION('ref_axis',(0.707106781186565,3.61482073326878E-14,-0.70710678118653));
#18004=DIRECTION('',(1.39941595733251E-14,-1.,1.66533453693773E-16));
#18005=DIRECTION('center_axis',(-0.707106781186545,2.27462860225727E-15,
-0.70710678118655));
#18006=DIRECTION('ref_axis',(0.70710678118655,-1.72044670028397E-13,-0.707106781186545));
#18007=DIRECTION('',(0.707106781186547,5.55111512312579E-17,-0.707106781186548));
#18008=DIRECTION('center_axis',(0.707106781186553,2.76828881917404E-14,
0.707106781186542));
#18009=DIRECTION('ref_axis',(0.707106781186542,1.08542133667551E-13,-0.707106781186553));
#18010=DIRECTION('',(6.98296272528204E-15,-1.,7.105427357601E-15));
#18011=DIRECTION('center_axis',(-2.64697796016969E-23,1.,1.66533453693773E-16));
#18012=DIRECTION('ref_axis',(2.64697796016969E-23,-1.66533453693774E-16,
1.));
#18013=DIRECTION('',(1.,-2.64697796016969E-23,2.64697796016969E-23));
#18014=DIRECTION('',(1.,-2.64697796016969E-23,2.64697796016969E-23));
#18015=DIRECTION('center_axis',(-2.64697796016969E-23,-1.66533453693773E-16,
-1.));
#18016=DIRECTION('ref_axis',(-2.64697796016969E-23,1.,-1.66533453693774E-16));
#18017=DIRECTION('',(1.,-2.64697796016969E-23,2.64697796016969E-23));
#18018=DIRECTION('center_axis',(5.29395592033937E-23,-1.,6.88338275267597E-15));
#18019=DIRECTION('ref_axis',(-5.29395592033938E-23,-6.88338275267597E-15,
-1.));
#18020=DIRECTION('',(1.,-2.64697796016969E-23,2.64697796016969E-23));
#18021=DIRECTION('center_axis',(1.,-2.64697796016969E-23,2.64697796016969E-23));
#18022=DIRECTION('ref_axis',(2.64697796016969E-23,-7.00649232162408E-46,
-1.));
#18023=DIRECTION('',(1.,-2.64697796016969E-23,2.64697796016969E-23));
#18024=DIRECTION('center_axis',(2.64697796016969E-23,1.66533453693773E-16,
1.));
#18025=DIRECTION('ref_axis',(2.64697796016969E-23,-1.,1.66533453693774E-16));
#18026=DIRECTION('',(1.,-2.64697796016969E-23,2.64697796016969E-23));
#18027=DIRECTION('center_axis',(1.,-2.64697796016969E-23,2.64697796016969E-23));
#18028=DIRECTION('ref_axis',(2.64697796016969E-23,-7.00649232162408E-46,
-1.));
#18029=DIRECTION('',(1.,-2.64697796016969E-23,2.64697796016969E-23));
#18030=DIRECTION('center_axis',(2.64697796016969E-23,-1.,-1.66533453693773E-16));
#18031=DIRECTION('ref_axis',(-2.64697796016969E-23,1.66533453693774E-16,
-1.));
#18032=DIRECTION('',(1.,-2.64697796016969E-23,2.64697796016969E-23));
#18033=DIRECTION('center_axis',(1.,-2.64697796016969E-23,2.64697796016969E-23));
#18034=DIRECTION('ref_axis',(2.64697796016969E-23,1.68147671338624E-16,
-1.));
#18035=DIRECTION('',(1.,-2.64697796016969E-23,2.64697796016969E-23));
#18036=DIRECTION('center_axis',(5.29395592033938E-23,7.105427357601E-15,
1.));
#18037=DIRECTION('ref_axis',(5.29395592033938E-23,-1.,7.105427357601E-15));
#18038=DIRECTION('center_axis',(1.16649072924818E-39,0.,1.));
#18039=DIRECTION('ref_axis',(1.,0.,-1.16649072924818E-39));
#18040=DIRECTION('center_axis',(1.16649072924818E-39,0.,1.));
#18041=DIRECTION('ref_axis',(1.,0.,-1.16649072924818E-39));
#18042=DIRECTION('',(1.16649072924818E-39,0.,1.));
#18043=DIRECTION('center_axis',(1.16649072924818E-39,0.,1.));
#18044=DIRECTION('ref_axis',(1.,-5.87747175411142E-39,-1.16649072924818E-39));
#18045=DIRECTION('center_axis',(1.16649072924818E-39,0.,1.));
#18046=DIRECTION('ref_axis',(-0.667534157816547,0.744579175204459,7.78672406549494E-40));
#18047=DIRECTION('center_axis',(1.16649072924818E-39,0.,1.));
#18048=DIRECTION('ref_axis',(1.,0.,-1.16649072924818E-39));
#18049=DIRECTION('',(1.16649072924818E-39,0.,1.));
#18050=DIRECTION('center_axis',(1.16649072924818E-39,0.,1.));
#18051=DIRECTION('ref_axis',(1.,-5.87747175411143E-39,-1.16649072924818E-39));
#18052=DIRECTION('',(1.16649072924818E-39,0.,1.));
#18053=DIRECTION('center_axis',(1.16649072924818E-39,0.,1.));
#18054=DIRECTION('ref_axis',(-0.744579175204457,-0.66753415781655,8.68544705067255E-40));
#18055=DIRECTION('center_axis',(-1.16649072924818E-39,0.,-1.));
#18056=DIRECTION('ref_axis',(-1.,0.,1.16649072924818E-39));
#18057=DIRECTION('',(1.16649072924818E-39,0.,1.));
#18058=DIRECTION('center_axis',(-1.16649072924818E-39,0.,-1.));
#18059=DIRECTION('ref_axis',(-1.,0.,1.16649072924818E-39));
#18060=DIRECTION('center_axis',(-1.44079214459515E-16,1.,0.));
#18061=DIRECTION('ref_axis',(-1.,-1.44079214459515E-16,1.43985447997384E-40));
#18062=DIRECTION('',(-1.,-1.44079214459515E-16,1.4398546441885E-40));
#18063=DIRECTION('',(1.16649072924818E-39,0.,1.));
#18064=DIRECTION('',(-1.,-1.44079214459515E-16,1.4398546441885E-40));
#18065=DIRECTION('center_axis',(0.707106781186544,0.707106781186551,0.));
#18066=DIRECTION('ref_axis',(-0.707106781186551,0.707106781186544,0.));
#18067=DIRECTION('',(-0.707106781186551,0.707106781186544,0.));
#18068=DIRECTION('',(1.16649072924818E-39,0.,1.));
#18069=DIRECTION('',(-0.707106781186551,0.707106781186544,0.));
#18070=DIRECTION('center_axis',(1.,-5.87747175411144E-39,-1.16649072924818E-39));
#18071=DIRECTION('ref_axis',(-1.16649072924818E-39,0.,-1.));
#18072=DIRECTION('',(-5.87747175411144E-39,1.,0.));
#18073=DIRECTION('',(1.16649072924818E-39,0.,1.));
#18074=DIRECTION('',(-5.87747175411144E-39,1.,0.));
#18075=DIRECTION('center_axis',(5.87747175411144E-39,-1.,-6.85601631258903E-78));
#18076=DIRECTION('ref_axis',(-1.16649072924818E-39,0.,-1.));
#18077=DIRECTION('',(1.,-5.87747175411144E-39,1.16649072924818E-39));
#18078=DIRECTION('',(1.,-5.87747175411144E-39,1.16649072924818E-39));
#18079=DIRECTION('center_axis',(-1.16649072924818E-39,1.37120326251781E-77,
1.));
#18080=DIRECTION('ref_axis',(1.,-5.87747175411144E-39,1.16649072924818E-39));
#18081=DIRECTION('center_axis',(-1.16649072924818E-39,1.37120326251781E-77,
1.));
#18082=DIRECTION('ref_axis',(1.,-5.87747175411144E-39,1.16649072924818E-39));
#18083=DIRECTION('center_axis',(-1.16649072924818E-39,0.,-1.));
#18084=DIRECTION('ref_axis',(-1.,0.,1.16649072924818E-39));
#18085=DIRECTION('center_axis',(1.16649072924818E-39,0.,1.));
#18086=DIRECTION('ref_axis',(1.,0.,-1.16649072924818E-39));
#18087=DIRECTION('',(-1.16649072924818E-39,0.,-1.));
#18088=DIRECTION('center_axis',(1.16649072924818E-39,0.,1.));
#18089=DIRECTION('ref_axis',(1.,0.,-1.16649072924818E-39));
#18090=DIRECTION('center_axis',(1.16649072924818E-39,-1.37120326251781E-77,
-1.));
#18091=DIRECTION('ref_axis',(-1.,5.87747175411144E-39,-1.16649072924818E-39));
#18092=DIRECTION('',(-0.707106781186682,-0.707106781186413,0.));
#18093=DIRECTION('',(5.87747175411144E-39,-1.,0.));
#18094=DIRECTION('',(1.,2.39272203583008E-16,5.10666202579846E-39));
#18095=DIRECTION('center_axis',(1.16649072924818E-39,0.,1.));
#18096=DIRECTION('ref_axis',(-1.,0.,1.16649072924818E-39));
#18097=DIRECTION('',(1.91417762866406E-15,1.,0.));
#18098=DIRECTION('',(-1.,2.16502149887901E-16,-9.40207082428935E-39));
#18099=DIRECTION('center_axis',(1.16649072924818E-39,-1.37120326251781E-77,
-1.));
#18100=DIRECTION('ref_axis',(-1.,5.87747175411144E-39,-1.16649072924818E-39));
#18101=DIRECTION('',(-0.707106781186682,-0.707106781186413,0.));
#18102=DIRECTION('',(-1.,2.16502149887901E-16,-9.40207082428935E-39));
#18103=DIRECTION('',(1.91417762866406E-15,1.,0.));
#18104=DIRECTION('center_axis',(1.16649072924818E-39,0.,1.));
#18105=DIRECTION('ref_axis',(-1.,0.,1.16649072924818E-39));
#18106=DIRECTION('',(1.,2.39272203583008E-16,5.10666202579846E-39));
#18107=DIRECTION('',(5.87747175411144E-39,-1.,0.));
#18108=DIRECTION('center_axis',(0.707106781186413,-0.707106781186682,0.));
#18109=DIRECTION('ref_axis',(0.707106781186682,0.707106781186413,0.));
#18110=DIRECTION('',(-1.16649072924818E-39,0.,-1.));
#18111=DIRECTION('',(-1.16649072924818E-39,0.,-1.));
#18112=DIRECTION('center_axis',(1.,-5.87747175411144E-39,-1.16649072924818E-39));
#18113=DIRECTION('ref_axis',(-1.16649072924818E-39,0.,-1.));
#18114=DIRECTION('',(-1.16649072924818E-39,0.,-1.));
#18115=DIRECTION('center_axis',(-2.39272203583008E-16,1.,0.));
#18116=DIRECTION('ref_axis',(-1.,-2.39272203583008E-16,-5.10666202579846E-39));
#18117=DIRECTION('',(-1.16649072924818E-39,0.,-1.));
#18118=DIRECTION('center_axis',(-1.16649072924818E-39,0.,-1.));
#18119=DIRECTION('ref_axis',(-1.,0.,1.16649072924818E-39));
#18120=DIRECTION('',(-1.16649072924818E-39,0.,-1.));
#18121=DIRECTION('center_axis',(-1.,1.91417762866406E-15,9.67520394012289E-40));
#18122=DIRECTION('ref_axis',(-1.91417762866406E-15,-1.,-7.68355080092362E-71));
#18123=DIRECTION('',(-1.16649072924818E-39,0.,-1.));
#18124=DIRECTION('center_axis',(-2.16502149887901E-16,-1.,0.));
#18125=DIRECTION('ref_axis',(1.,-2.16502149887901E-16,9.40207082428935E-39));
#18126=DIRECTION('center_axis',(-1.16649072924818E-39,0.,-1.));
#18127=DIRECTION('ref_axis',(1.,-8.81620763116713E-39,-1.16649072924818E-39));
#18128=DIRECTION('center_axis',(1.16649072924818E-39,0.,1.));
#18129=DIRECTION('ref_axis',(1.,-8.81620763116713E-39,-1.16649072924818E-39));
#18130=DIRECTION('',(-1.16649072924818E-39,0.,-1.));
#18131=DIRECTION('center_axis',(1.16649072924818E-39,0.,1.));
#18132=DIRECTION('ref_axis',(1.,-8.81620763116713E-39,-1.16649072924818E-39));
#18133=DIRECTION('center_axis',(-1.16649072924818E-39,0.,-1.));
#18134=DIRECTION('ref_axis',(-0.66753415781655,0.744579175204457,7.78672406549497E-40));
#18135=DIRECTION('center_axis',(1.16649072924818E-39,0.,1.));
#18136=DIRECTION('ref_axis',(1.,-8.81620763116715E-39,-1.16649072924818E-39));
#18137=DIRECTION('',(-1.16649072924818E-39,0.,-1.));
#18138=DIRECTION('center_axis',(1.16649072924818E-39,0.,1.));
#18139=DIRECTION('ref_axis',(1.,-8.81620763116715E-39,-1.16649072924818E-39));
#18140=DIRECTION('',(-1.16649072924818E-39,0.,-1.));
#18141=DIRECTION('center_axis',(-1.16649072924818E-39,0.,-1.));
#18142=DIRECTION('ref_axis',(-0.744579175204457,-0.66753415781655,8.68544705067255E-40));
#18143=DIRECTION('center_axis',(-1.16649072924818E-39,0.,-1.));
#18144=DIRECTION('ref_axis',(-1.,0.,1.16649072924818E-39));
#18145=DIRECTION('center_axis',(-1.16649072924818E-39,0.,-1.));
#18146=DIRECTION('ref_axis',(-1.,0.,1.16649072924818E-39));
#18147=DIRECTION('',(-1.16649072924818E-39,0.,-1.));
#18148=DIRECTION('center_axis',(-1.44079214459515E-16,1.,0.));
#18149=DIRECTION('ref_axis',(-1.,-1.44079214459515E-16,1.43985447997384E-40));
#18150=DIRECTION('',(-1.,-1.44079214459515E-16,1.4398546441885E-40));
#18151=DIRECTION('',(-1.,-1.44079214459515E-16,1.4398546441885E-40));
#18152=DIRECTION('',(-1.16649072924818E-39,0.,-1.));
#18153=DIRECTION('center_axis',(0.707106781186544,0.707106781186551,0.));
#18154=DIRECTION('ref_axis',(-0.707106781186551,0.707106781186544,0.));
#18155=DIRECTION('',(-0.707106781186551,0.707106781186544,0.));
#18156=DIRECTION('',(-0.707106781186551,0.707106781186544,0.));
#18157=DIRECTION('',(-1.16649072924818E-39,0.,-1.));
#18158=DIRECTION('center_axis',(1.,-8.81620763116716E-39,-1.16649072924818E-39));
#18159=DIRECTION('ref_axis',(1.16649072924818E-39,0.,1.));
#18160=DIRECTION('',(-8.81620763116716E-39,1.,0.));
#18161=DIRECTION('',(-8.81620763116716E-39,1.,0.));
#18162=DIRECTION('',(-1.16649072924818E-39,0.,-1.));
#18163=DIRECTION('center_axis',(8.81620763116716E-39,-1.,-1.02840244688835E-77));
#18164=DIRECTION('ref_axis',(1.16649072924818E-39,0.,1.));
#18165=DIRECTION('',(1.,-8.81620763116716E-39,1.16649072924818E-39));
#18166=DIRECTION('',(1.,-8.81620763116716E-39,1.16649072924818E-39));
#18167=DIRECTION('center_axis',(1.16649072924818E-39,-2.05680489377671E-77,
-1.));
#18168=DIRECTION('ref_axis',(1.,-8.81620763116716E-39,1.16649072924818E-39));
#18169=DIRECTION('center_axis',(1.16649072924818E-39,-2.05680489377671E-77,
-1.));
#18170=DIRECTION('ref_axis',(1.,-8.81620763116716E-39,1.16649072924818E-39));
#18171=DIRECTION('center_axis',(1.16649072924818E-39,0.,1.));
#18172=DIRECTION('ref_axis',(-1.,0.,1.16649072924818E-39));
#18173=DIRECTION('center_axis',(1.16649072924818E-39,0.,1.));
#18174=DIRECTION('ref_axis',(1.,0.,-1.16649072924818E-39));
#18175=DIRECTION('',(1.16649072924818E-39,0.,1.));
#18176=DIRECTION('center_axis',(1.16649072924818E-39,0.,1.));
#18177=DIRECTION('ref_axis',(1.,0.,-1.16649072924818E-39));
#18178=DIRECTION('center_axis',(-1.16649072924818E-39,2.05680489377671E-77,
1.));
#18179=DIRECTION('ref_axis',(-1.,8.81620763116716E-39,-1.16649072924818E-39));
#18180=DIRECTION('',(-0.707106781186682,-0.707106781186413,0.));
#18181=DIRECTION('',(-1.,2.16502149887901E-16,-4.4666901348958E-38));
#18182=DIRECTION('',(1.91417762866406E-15,1.,0.));
#18183=DIRECTION('center_axis',(1.16649072924818E-39,0.,1.));
#18184=DIRECTION('ref_axis',(-1.,0.,1.16649072924818E-39));
#18185=DIRECTION('',(1.,2.39272203583008E-16,2.27390772881328E-38));
#18186=DIRECTION('',(2.35098870164458E-38,-1.,0.));
#18187=DIRECTION('center_axis',(-1.16649072924818E-39,2.05680489377671E-77,
1.));
#18188=DIRECTION('ref_axis',(-1.,8.81620763116716E-39,-1.16649072924818E-39));
#18189=DIRECTION('',(-0.707106781186682,-0.707106781186413,0.));
#18190=DIRECTION('',(2.35098870164458E-38,-1.,0.));
#18191=DIRECTION('',(1.,2.39272203583008E-16,2.27390772881328E-38));
#18192=DIRECTION('center_axis',(1.16649072924818E-39,0.,1.));
#18193=DIRECTION('ref_axis',(-1.,0.,1.16649072924818E-39));
#18194=DIRECTION('',(1.91417762866406E-15,1.,0.));
#18195=DIRECTION('',(-1.,2.16502149887901E-16,-4.4666901348958E-38));
#18196=DIRECTION('center_axis',(0.707106781186413,-0.707106781186682,0.));
#18197=DIRECTION('ref_axis',(0.707106781186682,0.707106781186413,0.));
#18198=DIRECTION('',(1.16649072924818E-39,0.,1.));
#18199=DIRECTION('',(1.16649072924818E-39,0.,1.));
#18200=DIRECTION('center_axis',(1.,-8.81620763116716E-39,-1.16649072924818E-39));
#18201=DIRECTION('ref_axis',(1.16649072924818E-39,0.,1.));
#18202=DIRECTION('',(1.16649072924818E-39,0.,1.));
#18203=DIRECTION('center_axis',(-2.39272203583008E-16,1.,0.));
#18204=DIRECTION('ref_axis',(-1.,-2.39272203583008E-16,-2.27390772881328E-38));
#18205=DIRECTION('',(1.16649072924818E-39,0.,1.));
#18206=DIRECTION('center_axis',(1.16649072924818E-39,0.,1.));
#18207=DIRECTION('ref_axis',(-1.,0.,1.16649072924818E-39));
#18208=DIRECTION('',(1.16649072924818E-39,0.,1.));
#18209=DIRECTION('center_axis',(-1.,1.91417762866406E-15,9.67520394012289E-40));
#18210=DIRECTION('ref_axis',(-1.91417762866406E-15,-1.,-7.68355080092362E-71));
#18211=DIRECTION('',(1.16649072924818E-39,0.,1.));
#18212=DIRECTION('center_axis',(-2.16502149887901E-16,-1.,0.));
#18213=DIRECTION('ref_axis',(1.,-2.16502149887901E-16,4.4666901348958E-38));
#18214=DIRECTION('center_axis',(7.04991620636974E-15,1.,0.));
#18215=DIRECTION('ref_axis',(-1.,7.04991620636974E-15,0.));
#18216=DIRECTION('center_axis',(-6.96737689119829E-15,-1.,0.));
#18217=DIRECTION('ref_axis',(1.,-6.96737689119829E-15,0.));
#18218=DIRECTION('',(7.04991620636974E-15,1.,0.));
#18219=DIRECTION('center_axis',(7.04991620636974E-15,1.,0.));
#18220=DIRECTION('ref_axis',(-1.,7.04991620636974E-15,0.));
#18221=DIRECTION('',(7.04991620636974E-15,1.,0.));
#18222=DIRECTION('center_axis',(7.04991620636974E-15,1.,0.));
#18223=DIRECTION('ref_axis',(-1.,7.04991620636974E-15,0.));
#18224=DIRECTION('center_axis',(-6.96737689119829E-15,-1.,0.));
#18225=DIRECTION('ref_axis',(1.,-6.96737689119829E-15,0.));
#18226=DIRECTION('',(7.04991620636974E-15,1.,0.));
#18227=DIRECTION('center_axis',(7.04991620636974E-15,1.,0.));
#18228=DIRECTION('ref_axis',(-1.,7.04991620636974E-15,0.));
#18229=DIRECTION('',(7.04991620636974E-15,1.,0.));
#18230=DIRECTION('center_axis',(-1.16649072924818E-39,0.,-1.));
#18231=DIRECTION('ref_axis',(-1.,0.,1.16649072924818E-39));
#18232=DIRECTION('center_axis',(-1.16649072924818E-39,0.,-1.));
#18233=DIRECTION('ref_axis',(1.,-7.10423911405687E-15,-1.16649072924818E-39));
#18234=DIRECTION('',(-1.16649072924818E-39,0.,-1.));
#18235=DIRECTION('center_axis',(1.16649072924818E-39,0.,1.));
#18236=DIRECTION('ref_axis',(-1.,0.,1.16649072924818E-39));
#18237=DIRECTION('',(-1.16649072924818E-39,0.,-1.));
#18238=DIRECTION('center_axis',(-1.16649072924818E-39,0.,-1.));
#18239=DIRECTION('ref_axis',(-1.,0.,1.16649072924818E-39));
#18240=DIRECTION('center_axis',(-1.16649072924818E-39,0.,-1.));
#18241=DIRECTION('ref_axis',(1.,-7.10423911405687E-15,-1.16649072924818E-39));
#18242=DIRECTION('',(-1.16649072924818E-39,0.,-1.));
#18243=DIRECTION('center_axis',(0.707106781186548,0.,-0.707106781186548));
#18244=DIRECTION('ref_axis',(0.707106781186548,2.39812798898023E-13,0.707106781186548));
#18245=DIRECTION('',(-1.16649072924818E-39,0.,-1.));
#18246=DIRECTION('center_axis',(1.,-5.87747175411144E-39,-1.16649072924818E-39));
#18247=DIRECTION('ref_axis',(-1.16649072924818E-39,0.,-1.));
#18248=DIRECTION('',(5.87747175411144E-39,-1.,0.));
#18249=DIRECTION('',(-1.16649072924818E-39,0.,-1.));
#18250=DIRECTION('',(-5.87747175411144E-39,1.,0.));
#18251=DIRECTION('center_axis',(1.,-5.87747175411144E-39,-1.16649072924818E-39));
#18252=DIRECTION('ref_axis',(-1.16649072924818E-39,0.,-1.));
#18253=DIRECTION('',(5.87747175411144E-39,-1.,0.));
#18254=DIRECTION('',(-1.16649072924818E-39,0.,-1.));
#18255=DIRECTION('',(5.87747175411144E-39,-1.,-6.98296267768627E-15));
#18256=DIRECTION('center_axis',(-0.707106781186547,4.93770026216453E-15,
-0.707106781186548));
#18257=DIRECTION('ref_axis',(-0.707106781186548,7.14278800091209E-32,0.707106781186547));
#18258=DIRECTION('',(-5.87747175411144E-39,1.,6.98296267768627E-15));
#18259=DIRECTION('center_axis',(0.707106781186551,-7.63665881151437E-15,
0.707106781186544));
#18260=DIRECTION('ref_axis',(0.707106781186544,-1.83022781783008E-13,-0.707106781186551));
#18261=DIRECTION('',(0.707106781186548,-4.92667944684876E-15,-0.707106781186548));
#18262=DIRECTION('center_axis',(-0.707106781186549,5.37639487806273E-15,
-0.707106781186546));
#18263=DIRECTION('ref_axis',(0.707106781186546,-2.782375660343E-13,-0.707106781186549));
#18264=DIRECTION('',(7.01119687164608E-15,1.,-2.82341939598112E-17));
#18265=DIRECTION('center_axis',(0.70710678118654,1.56975764458913E-14,0.707106781186555));
#18266=DIRECTION('ref_axis',(0.707106781186555,4.95830950211E-13,-0.70710678118654));
#18267=DIRECTION('',(0.707106781186548,0.,-0.707106781186548));
#18268=DIRECTION('',(-7.02672800395669E-15,-1.,4.37653262704196E-17));
#18269=DIRECTION('',(-0.707106781186548,4.93770026216453E-15,0.707106781186548));
#18270=DIRECTION('center_axis',(-0.707106781186547,-4.93770026216453E-15,
0.707106781186548));
#18271=DIRECTION('ref_axis',(0.707106781186548,1.39101446851167E-31,0.707106781186547));
#18272=DIRECTION('',(0.707106781186548,-4.93770026216453E-15,0.707106781186548));
#18273=DIRECTION('',(7.02672800395669E-15,1.,1.4009690681643E-14));
#18274=DIRECTION('',(-0.707106781186548,0.,-0.707106781186547));
#18275=DIRECTION('center_axis',(0.707106781186553,-4.56078234576569E-15,
-0.707106781186542));
#18276=DIRECTION('ref_axis',(0.707106781186542,3.97390229061337E-13,0.707106781186553));
#18277=DIRECTION('',(-7.01119687164608E-15,-1.,-1.39941595493323E-14));
#18278=DIRECTION('center_axis',(-0.707106781186546,-5.37639487806278E-15,
0.707106781186549));
#18279=DIRECTION('ref_axis',(0.707106781186549,-5.8955593170548E-14,0.707106781186546));
#18280=DIRECTION('',(-0.707106781186548,4.92667944684876E-15,-0.707106781186548));
#18281=DIRECTION('center_axis',(6.98296267768627E-15,1.,0.));
#18282=DIRECTION('ref_axis',(-1.,6.98296267768627E-15,-1.76663133728356E-39));
#18283=DIRECTION('',(1.,-7.04991620636974E-15,-8.33232385715269E-40));
#18284=DIRECTION('',(-1.,7.04991620636974E-15,8.33232385715269E-40));
#18285=DIRECTION('',(-1.16649072924818E-39,0.,-1.));
#18286=DIRECTION('',(-1.16649072924818E-39,0.,-1.));
#18287=DIRECTION('',(1.,-7.04991620636974E-15,-8.33232385715269E-40));
#18288=DIRECTION('',(-1.,7.04991620636974E-15,8.33232385715269E-40));
#18289=DIRECTION('center_axis',(-1.,7.02672800395669E-15,-2.86337824953972E-41));
#18290=DIRECTION('ref_axis',(-7.02672800395669E-15,-1.,-1.7794652584401E-71));
#18291=DIRECTION('',(-1.16649072924818E-39,0.,-1.));
#18292=DIRECTION('center_axis',(5.87747175411144E-39,-1.,-6.85601631258903E-78));
#18293=DIRECTION('ref_axis',(-1.16649072924818E-39,0.,-1.));
#18294=DIRECTION('',(-1.16649072924818E-39,0.,-1.));
#18295=DIRECTION('center_axis',(-1.16649072924818E-39,0.,-1.));
#18296=DIRECTION('ref_axis',(-1.,0.,1.16649072924818E-39));
#18297=DIRECTION('',(-1.16649072924818E-39,0.,-1.));
#18298=DIRECTION('center_axis',(1.,-7.01119687164608E-15,1.79234866735008E-39));
#18299=DIRECTION('ref_axis',(7.01119687164608E-15,1.,-4.81896270872514E-70));
#18300=DIRECTION('',(-1.16649072924818E-39,0.,-1.));
#18301=DIRECTION('center_axis',(-1.16649072924818E-39,0.,-1.));
#18302=DIRECTION('ref_axis',(-1.,0.,1.16649072924818E-39));
#18303=DIRECTION('',(-1.16649072924818E-39,0.,-1.));
#18304=DIRECTION('center_axis',(-6.96737689119829E-15,-1.,0.));
#18305=DIRECTION('ref_axis',(1.,-6.96737689119829E-15,-1.58475996252038E-40));
#18306=DIRECTION('',(-1.,6.96737689119829E-15,1.58475996252038E-40));
#18307=DIRECTION('',(1.,-6.96737689119829E-15,-1.58475996252038E-40));
#18308=DIRECTION('',(-1.,6.96737689119829E-15,1.58475996252038E-40));
#18309=DIRECTION('',(-1.16649072924818E-39,0.,-1.));
#18310=DIRECTION('',(1.,-6.96737689119829E-15,-1.58475996252038E-40));
#18311=DIRECTION('center_axis',(-1.16649072924818E-39,0.,-1.));
#18312=DIRECTION('ref_axis',(-1.,0.,1.16649072924818E-39));
#18313=DIRECTION('center_axis',(1.16649072924818E-39,0.,1.));
#18314=DIRECTION('ref_axis',(-1.,0.,1.16649072924818E-39));
#18315=DIRECTION('',(-1.16649072924818E-39,0.,-1.));
#18316=DIRECTION('center_axis',(1.,-5.87747175411144E-39,-1.16649072924818E-39));
#18317=DIRECTION('ref_axis',(-1.16649072924818E-39,0.,-1.));
#18318=DIRECTION('',(-5.87747175411144E-39,1.,0.));
#18319=DIRECTION('center_axis',(-1.16649072924818E-39,1.37120326251781E-77,
1.));
#18320=DIRECTION('ref_axis',(1.,-5.87747175411144E-39,1.16649072924818E-39));
#18321=DIRECTION('center_axis',(1.16649072924818E-39,-1.37120326251781E-77,
-1.));
#18322=DIRECTION('ref_axis',(-1.,5.87747175411144E-39,-1.16649072924818E-39));
#18323=DIRECTION('center_axis',(-1.16649072924818E-39,1.37120326251781E-77,
1.));
#18324=DIRECTION('ref_axis',(1.,-5.87747175411144E-39,1.16649072924818E-39));
#18325=DIRECTION('center_axis',(1.16649072924818E-39,-1.37120326251781E-77,
-1.));
#18326=DIRECTION('ref_axis',(-1.,5.87747175411144E-39,-1.16649072924818E-39));
#18327=DIRECTION('center_axis',(1.16649072924818E-39,0.,1.));
#18328=DIRECTION('ref_axis',(-1.,0.,1.16649072924818E-39));
#18329=DIRECTION('center_axis',(1.16649072924818E-39,0.,1.));
#18330=DIRECTION('ref_axis',(1.,0.,-1.16649072924818E-39));
#18331=DIRECTION('',(1.16649072924818E-39,0.,1.));
#18332=DIRECTION('center_axis',(1.16649072924818E-39,0.,1.));
#18333=DIRECTION('ref_axis',(1.,0.,-1.16649072924818E-39));
#18334=DIRECTION('center_axis',(-1.16649072924818E-39,1.37120326251781E-77,
1.));
#18335=DIRECTION('ref_axis',(-1.,5.87747175411144E-39,-1.16649072924818E-39));
#18336=DIRECTION('',(-0.707106781186682,-0.707106781186413,0.));
#18337=DIRECTION('',(-1.,2.16502149887901E-16,-9.40207082428935E-39));
#18338=DIRECTION('',(1.91417762866406E-15,1.,0.));
#18339=DIRECTION('center_axis',(1.16649072924818E-39,0.,1.));
#18340=DIRECTION('ref_axis',(-1.,0.,1.16649072924818E-39));
#18341=DIRECTION('',(1.,2.39272203583008E-16,5.10666202579846E-39));
#18342=DIRECTION('',(5.87747175411144E-39,-1.,0.));
#18343=DIRECTION('center_axis',(-1.16649072924818E-39,1.37120326251781E-77,
1.));
#18344=DIRECTION('ref_axis',(-1.,5.87747175411144E-39,-1.16649072924818E-39));
#18345=DIRECTION('',(-0.707106781186682,-0.707106781186413,0.));
#18346=DIRECTION('',(5.87747175411144E-39,-1.,0.));
#18347=DIRECTION('',(1.,2.39272203583008E-16,5.10666202579846E-39));
#18348=DIRECTION('center_axis',(1.16649072924818E-39,0.,1.));
#18349=DIRECTION('ref_axis',(-1.,0.,1.16649072924818E-39));
#18350=DIRECTION('',(1.91417762866406E-15,1.,0.));
#18351=DIRECTION('',(-1.,2.16502149887901E-16,-9.40207082428935E-39));
#18352=DIRECTION('center_axis',(0.707106781186413,-0.707106781186682,0.));
#18353=DIRECTION('ref_axis',(0.707106781186682,0.707106781186413,0.));
#18354=DIRECTION('',(1.16649072924818E-39,0.,1.));
#18355=DIRECTION('',(1.16649072924818E-39,0.,1.));
#18356=DIRECTION('center_axis',(1.,-5.87747175411144E-39,-1.16649072924818E-39));
#18357=DIRECTION('ref_axis',(1.16649072924818E-39,0.,1.));
#18358=DIRECTION('',(1.16649072924818E-39,0.,1.));
#18359=DIRECTION('center_axis',(-2.39272203583008E-16,1.,0.));
#18360=DIRECTION('ref_axis',(-1.,-2.39272203583008E-16,-5.10666202579846E-39));
#18361=DIRECTION('',(1.16649072924818E-39,0.,1.));
#18362=DIRECTION('center_axis',(1.16649072924818E-39,0.,1.));
#18363=DIRECTION('ref_axis',(-1.,0.,1.16649072924818E-39));
#18364=DIRECTION('',(1.16649072924818E-39,0.,1.));
#18365=DIRECTION('center_axis',(-1.,1.91417762866406E-15,9.67520394012289E-40));
#18366=DIRECTION('ref_axis',(-1.91417762866406E-15,-1.,-7.68355080092362E-71));
#18367=DIRECTION('',(1.16649072924818E-39,0.,1.));
#18368=DIRECTION('center_axis',(-2.16502149887901E-16,-1.,0.));
#18369=DIRECTION('ref_axis',(1.,-2.16502149887901E-16,9.40207082428935E-39));
#18370=DIRECTION('center_axis',(-1.16649072924818E-39,0.,-1.));
#18371=DIRECTION('ref_axis',(-1.,0.,1.16649072924818E-39));
#18372=DIRECTION('center_axis',(1.16649072924818E-39,0.,1.));
#18373=DIRECTION('ref_axis',(1.,0.,-1.16649072924818E-39));
#18374=DIRECTION('',(-1.16649072924818E-39,0.,-1.));
#18375=DIRECTION('center_axis',(1.16649072924818E-39,0.,1.));
#18376=DIRECTION('ref_axis',(1.,0.,-1.16649072924818E-39));
#18377=DIRECTION('center_axis',(1.16649072924818E-39,-1.37120326251781E-77,
-1.));
#18378=DIRECTION('ref_axis',(-1.,5.87747175411144E-39,-1.16649072924818E-39));
#18379=DIRECTION('',(-0.707106781186682,-0.707106781186413,0.));
#18380=DIRECTION('',(5.87747175411144E-39,-1.,0.));
#18381=DIRECTION('',(1.,2.39272203583008E-16,5.10666202579846E-39));
#18382=DIRECTION('center_axis',(1.16649072924818E-39,0.,1.));
#18383=DIRECTION('ref_axis',(-1.,0.,1.16649072924818E-39));
#18384=DIRECTION('',(1.91417762866406E-15,1.,0.));
#18385=DIRECTION('',(-1.,2.16502149887901E-16,-9.40207082428935E-39));
#18386=DIRECTION('center_axis',(1.16649072924818E-39,-1.37120326251781E-77,
-1.));
#18387=DIRECTION('ref_axis',(-1.,5.87747175411144E-39,-1.16649072924818E-39));
#18388=DIRECTION('',(-0.707106781186682,-0.707106781186413,0.));
#18389=DIRECTION('',(-1.,2.16502149887901E-16,-9.40207082428935E-39));
#18390=DIRECTION('',(1.91417762866406E-15,1.,0.));
#18391=DIRECTION('center_axis',(1.16649072924818E-39,0.,1.));
#18392=DIRECTION('ref_axis',(-1.,0.,1.16649072924818E-39));
#18393=DIRECTION('',(1.,2.39272203583008E-16,5.10666202579846E-39));
#18394=DIRECTION('',(5.87747175411144E-39,-1.,0.));
#18395=DIRECTION('center_axis',(0.707106781186413,-0.707106781186682,0.));
#18396=DIRECTION('ref_axis',(0.707106781186682,0.707106781186413,0.));
#18397=DIRECTION('',(-1.16649072924818E-39,0.,-1.));
#18398=DIRECTION('',(-1.16649072924818E-39,0.,-1.));
#18399=DIRECTION('center_axis',(1.,-5.87747175411144E-39,-1.16649072924818E-39));
#18400=DIRECTION('ref_axis',(-1.16649072924818E-39,0.,-1.));
#18401=DIRECTION('',(-1.16649072924818E-39,0.,-1.));
#18402=DIRECTION('center_axis',(-2.39272203583008E-16,1.,0.));
#18403=DIRECTION('ref_axis',(-1.,-2.39272203583008E-16,-5.10666202579846E-39));
#18404=DIRECTION('',(-1.16649072924818E-39,0.,-1.));
#18405=DIRECTION('center_axis',(-1.16649072924818E-39,0.,-1.));
#18406=DIRECTION('ref_axis',(-1.,0.,1.16649072924818E-39));
#18407=DIRECTION('',(-1.16649072924818E-39,0.,-1.));
#18408=DIRECTION('center_axis',(-1.,1.91417762866406E-15,9.67520394012289E-40));
#18409=DIRECTION('ref_axis',(-1.91417762866406E-15,-1.,-7.68355080092362E-71));
#18410=DIRECTION('',(-1.16649072924818E-39,0.,-1.));
#18411=DIRECTION('center_axis',(-2.16502149887901E-16,-1.,0.));
#18412=DIRECTION('ref_axis',(1.,-2.16502149887901E-16,9.40207082428935E-39));
#21977=CARTESIAN_POINT('',(0.,0.,0.));
#21978=CARTESIAN_POINT('Origin',(-250.,0.,-200.));
#21979=CARTESIAN_POINT('',(-313.2,1.11022302462516E-13,-263.2));
#21980=CARTESIAN_POINT('',(-313.2,-0.199999999999922,-263.2));
#21981=CARTESIAN_POINT('',(-313.2,-3.33066907387547E-13,-263.2));
#21982=CARTESIAN_POINT('',(-250.,0.,-200.));
#21983=CARTESIAN_POINT('',(-281.6,1.11022302462516E-13,-231.6));
#21984=CARTESIAN_POINT('',(-250.,-63.2,-199.999999999999));
#21985=CARTESIAN_POINT('',(-250.,0.,-200.));
#21986=CARTESIAN_POINT('',(-250.2,-63.2,-200.2));
#21987=CARTESIAN_POINT('',(-250.,-63.2,-200.));
#21988=CARTESIAN_POINT('',(-257.9375,-55.4625,-207.937499999999));
#21989=CARTESIAN_POINT('Origin',(-250.199999999997,-55.4624999999972,-200.199999999997));
#21990=CARTESIAN_POINT('',(-257.9375,-15.875,-207.9375));
#21991=CARTESIAN_POINT('',(-257.9375,-55.4625000000001,-207.937499999999));
#21992=CARTESIAN_POINT('',(-265.875,-7.93749999999999,-215.875));
#21993=CARTESIAN_POINT('Origin',(-265.875000000001,-15.875000000001,-215.875000000001));
#21994=CARTESIAN_POINT('',(-305.4625,-7.93749999999988,-255.4625));
#21995=CARTESIAN_POINT('',(-257.9375,-7.93749999999999,-207.9375));
#21996=CARTESIAN_POINT('Origin',(-305.462499999999,-0.199999999998104,-255.462499999999));
#21997=CARTESIAN_POINT('Origin',(-250.,0.,200.));
#21998=CARTESIAN_POINT('',(-313.2,0.,263.2));
#21999=CARTESIAN_POINT('',(-250.,0.,200.));
#22000=CARTESIAN_POINT('',(-81.5999999999998,0.,31.5999999999999));
#22001=CARTESIAN_POINT('',(-313.2,-0.199999999999978,263.2));
#22002=CARTESIAN_POINT('',(-313.2,9.71445146547012E-12,263.2));
#22003=CARTESIAN_POINT('',(-305.4625,-7.93749999999999,255.4625));
#22004=CARTESIAN_POINT('Origin',(-305.462500000002,-0.200000000002175,255.462500000002));
#22005=CARTESIAN_POINT('',(-265.875,-7.93749999999999,215.875));
#22006=CARTESIAN_POINT('',(-57.9374999999998,-7.93749999999999,7.93749999999999));
#22007=CARTESIAN_POINT('',(-257.9375,-15.875,207.9375));
#22008=CARTESIAN_POINT('Origin',(-265.875000000001,-15.8750000000013,215.875000000002));
#22009=CARTESIAN_POINT('',(-257.9375,-55.4625,207.937500000001));
#22010=CARTESIAN_POINT('',(-257.9375,-55.4624999999943,207.937500000001));
#22011=CARTESIAN_POINT('',(-250.2,-63.2,200.200000000001));
#22012=CARTESIAN_POINT('Origin',(-250.2,-55.4625000000004,200.200000000001));
#22013=CARTESIAN_POINT('',(-250.,-63.2,200.000000000001));
#22014=CARTESIAN_POINT('',(-49.9999999999996,-63.2000000000014,5.55111512312578E-13));
#22015=CARTESIAN_POINT('',(-250.,5.55111512312578E-12,200.));
#22016=CARTESIAN_POINT('Origin',(-313.2,0.,-200.));
#22017=CARTESIAN_POINT('',(-250.,0.,-200.));
#22018=CARTESIAN_POINT('',(-313.2,0.,-200.));
#22019=CARTESIAN_POINT('Origin',(-250.,0.,-200.));
#22020=CARTESIAN_POINT('',(-250.,-63.2,-200.));
#22021=CARTESIAN_POINT('Origin',(-250.,-63.2,-200.));
#22022=CARTESIAN_POINT('',(-250.2,-63.2,-200.));
#22023=CARTESIAN_POINT('Origin',(-250.2,-55.4625,-200.));
#22024=CARTESIAN_POINT('',(-257.9375,-55.4625,-200.));
#22025=CARTESIAN_POINT('Origin',(-257.9375,-55.4625,-200.));
#22026=CARTESIAN_POINT('',(-257.9375,-15.875,-200.));
#22027=CARTESIAN_POINT('Origin',(-265.875,-15.875,-200.));
#22028=CARTESIAN_POINT('',(-265.875,-7.93749999999999,-200.));
#22029=CARTESIAN_POINT('Origin',(-265.875,-7.93749999999999,-200.));
#22030=CARTESIAN_POINT('',(-305.4625,-7.93749999999999,-200.));
#22031=CARTESIAN_POINT('Origin',(-305.4625,-0.199999999999978,-200.));
#22032=CARTESIAN_POINT('',(-313.2,-0.199999999999978,-200.));
#22033=CARTESIAN_POINT('Origin',(-313.2,0.,-200.));
#22034=CARTESIAN_POINT('Origin',(-250.,0.,-200.));
#22035=CARTESIAN_POINT('',(-313.2,-0.199999999999922,-263.2));
#22036=CARTESIAN_POINT('',(-313.2,1.11022302462516E-13,-263.2));
#22037=CARTESIAN_POINT('',(-313.2,1.18793863634892E-11,-263.2));
#22038=CARTESIAN_POINT('',(-305.4625,-7.93749999999988,-255.4625));
#22039=CARTESIAN_POINT('Origin',(-305.4625,-0.19999999999989,-255.4625));
#22040=CARTESIAN_POINT('',(-265.875,-7.93749999999999,-215.875));
#22041=CARTESIAN_POINT('',(-7.93749999999999,-7.93749999999999,42.0625000000001));
#22042=CARTESIAN_POINT('',(-257.9375,-15.875,-207.9375));
#22043=CARTESIAN_POINT('Origin',(-265.875000000001,-15.8750000000005,-215.875000000001));
#22044=CARTESIAN_POINT('',(-257.937500000001,-55.4625,-207.9375));
#22045=CARTESIAN_POINT('',(-257.937500000001,-55.4624999999929,-207.9375));
#22046=CARTESIAN_POINT('',(-250.200000000001,-63.2,-200.2));
#22047=CARTESIAN_POINT('Origin',(-250.200000000001,-55.4624999999997,-200.2));
#22048=CARTESIAN_POINT('',(-250.000000000001,-63.2,-200.));
#22049=CARTESIAN_POINT('',(-4.99600519899998E-13,-63.2000000000018,50.0000000000003));
#22050=CARTESIAN_POINT('',(-250.,0.,-200.));
#22051=CARTESIAN_POINT('',(-250.,6.93889390390723E-12,-200.));
#22052=CARTESIAN_POINT('',(-31.5999999999999,0.,18.4000000000001));
#22053=CARTESIAN_POINT('Origin',(250.,0.,-200.));
#22054=CARTESIAN_POINT('',(250.,0.,-200.));
#22055=CARTESIAN_POINT('',(313.2,1.11022302462516E-13,-263.2));
#22056=CARTESIAN_POINT('',(281.6,1.11022302462516E-13,-231.6));
#22057=CARTESIAN_POINT('',(250.,-63.2,-200.));
#22058=CARTESIAN_POINT('',(250.,0.,-200.));
#22059=CARTESIAN_POINT('',(250.2,-63.2,-200.2));
#22060=CARTESIAN_POINT('',(250.,-63.2,-200.));
#22061=CARTESIAN_POINT('',(257.9375,-55.4625,-207.9375));
#22062=CARTESIAN_POINT('Origin',(250.200000000001,-55.4625000000011,-200.200000000001));
#22063=CARTESIAN_POINT('',(257.9375,-15.875,-207.9375));
#22064=CARTESIAN_POINT('',(257.9375,-55.4625000000001,-207.9375));
#22065=CARTESIAN_POINT('',(265.875,-7.93749999999999,-215.875));
#22066=CARTESIAN_POINT('Origin',(265.874999999997,-15.8749999999967,-215.874999999997));
#22067=CARTESIAN_POINT('',(305.4625,-7.93749999999988,-255.4625));
#22068=CARTESIAN_POINT('',(257.9375,-7.93749999999999,-207.9375));
#22069=CARTESIAN_POINT('',(313.2,-0.199999999999867,-263.2));
#22070=CARTESIAN_POINT('Origin',(305.4625,-0.199999999999467,-255.4625));
#22071=CARTESIAN_POINT('',(313.2,1.11022302462516E-13,-263.2));
#22072=CARTESIAN_POINT('Origin',(250.,1.11022302462516E-13,-263.2));
#22073=CARTESIAN_POINT('',(250.,1.11022302462516E-13,-263.2));
#22074=CARTESIAN_POINT('',(250.,0.,-200.));
#22075=CARTESIAN_POINT('Origin',(250.,0.,-200.));
#22076=CARTESIAN_POINT('',(250.,-63.2,-200.));
#22077=CARTESIAN_POINT('Origin',(250.,-63.2,-200.));
#22078=CARTESIAN_POINT('',(250.,-63.2,-200.2));
#22079=CARTESIAN_POINT('Origin',(250.,-55.4625,-200.2));
#22080=CARTESIAN_POINT('',(250.,-55.4625,-207.9375));
#22081=CARTESIAN_POINT('Origin',(250.,-55.4625,-207.9375));
#22082=CARTESIAN_POINT('',(250.,-15.875,-207.9375));
#22083=CARTESIAN_POINT('Origin',(250.,-15.875,-215.875));
#22084=CARTESIAN_POINT('',(250.,-7.93749999999999,-215.875));
#22085=CARTESIAN_POINT('Origin',(250.,-7.93749999999999,-215.875));
#22086=CARTESIAN_POINT('',(250.,-7.93749999999993,-255.4625));
#22087=CARTESIAN_POINT('Origin',(250.,-0.199999999999922,-255.4625));
#22088=CARTESIAN_POINT('',(250.,-0.199999999999922,-263.2));
#22089=CARTESIAN_POINT('Origin',(250.,1.11022302462516E-13,-263.2));
#22090=CARTESIAN_POINT('Origin',(250.,0.,200.));
#22091=CARTESIAN_POINT('',(313.2,-0.199999999999978,263.2));
#22092=CARTESIAN_POINT('',(313.2,0.,263.2));
#22093=CARTESIAN_POINT('',(313.2,7.88258347483861E-12,263.2));
#22094=CARTESIAN_POINT('',(305.4625,-7.93749999999999,255.4625));
#22095=CARTESIAN_POINT('Origin',(305.462500000003,-0.200000000002943,255.462500000003));
#22096=CARTESIAN_POINT('',(265.875,-7.93749999999999,215.875));
#22097=CARTESIAN_POINT('',(7.93749999999993,-7.93749999999988,-42.0625));
#22098=CARTESIAN_POINT('',(257.9375,-15.875,207.9375));
#22099=CARTESIAN_POINT('Origin',(265.874999999999,-15.8749999999993,215.874999999999));
#22100=CARTESIAN_POINT('',(257.9375,-55.4625,207.9375));
#22101=CARTESIAN_POINT('',(257.9375,-55.4624999999965,207.9375));
#22102=CARTESIAN_POINT('',(250.2,-63.2,200.2));
#22103=CARTESIAN_POINT('Origin',(250.200000000001,-55.4625000000004,200.200000000001));
#22104=CARTESIAN_POINT('',(250.,-63.2,200.));
#22105=CARTESIAN_POINT('',(3.88578111558364E-13,-63.2000000000016,-50.));
#22106=CARTESIAN_POINT('',(250.,0.,200.));
#22107=CARTESIAN_POINT('',(250.,3.49720252756924E-12,200.));
#22108=CARTESIAN_POINT('',(31.5999999999999,5.55111512312578E-14,-18.4));
#22109=CARTESIAN_POINT('Origin',(-250.,0.,200.));
#22110=CARTESIAN_POINT('',(-250.,0.,200.));
#22111=CARTESIAN_POINT('',(-313.2,0.,263.2));
#22112=CARTESIAN_POINT('',(-281.6,0.,231.6));
#22113=CARTESIAN_POINT('',(-250.,-63.2,200.));
#22114=CARTESIAN_POINT('',(-250.,0.,200.));
#22115=CARTESIAN_POINT('',(-250.199999999999,-63.2,200.2));
#22116=CARTESIAN_POINT('',(-250.,-63.2,200.));
#22117=CARTESIAN_POINT('',(-257.937499999999,-55.4625,207.9375));
#22118=CARTESIAN_POINT('Origin',(-250.199999999999,-55.4624999999993,200.2));
#22119=CARTESIAN_POINT('',(-257.9375,-15.875,207.9375));
#22120=CARTESIAN_POINT('',(-257.937499999999,-55.4625000000001,207.9375));
#22121=CARTESIAN_POINT('',(-265.875,-7.93749999999999,215.875));
#22122=CARTESIAN_POINT('Origin',(-265.874999999999,-15.8749999999987,215.874999999999));
#22123=CARTESIAN_POINT('',(-305.4625,-7.93749999999999,255.4625));
#22124=CARTESIAN_POINT('',(-257.9375,-7.93749999999999,207.9375));
#22125=CARTESIAN_POINT('',(-313.2,-0.199999999999978,263.2));
#22126=CARTESIAN_POINT('Origin',(-305.462499999999,-0.199999999999151,255.462499999999));
#22127=CARTESIAN_POINT('',(-313.2,-4.44089209850063E-13,263.2));
#22128=CARTESIAN_POINT('Origin',(-250.,0.,263.2));
#22129=CARTESIAN_POINT('',(-250.,0.,263.2));
#22130=CARTESIAN_POINT('',(-250.,0.,200.));
#22131=CARTESIAN_POINT('Origin',(-250.,0.,200.));
#22132=CARTESIAN_POINT('',(-250.,-63.2,200.));
#22133=CARTESIAN_POINT('Origin',(-250.,-63.2,200.));
#22134=CARTESIAN_POINT('',(-250.,-63.2,200.2));
#22135=CARTESIAN_POINT('Origin',(-250.,-55.4625,200.2));
#22136=CARTESIAN_POINT('',(-250.,-55.4625,207.9375));
#22137=CARTESIAN_POINT('Origin',(-250.,-55.4625,207.9375));
#22138=CARTESIAN_POINT('',(-250.,-15.875,207.9375));
#22139=CARTESIAN_POINT('Origin',(-250.,-15.875,215.875));
#22140=CARTESIAN_POINT('',(-250.,-7.93749999999999,215.875));
#22141=CARTESIAN_POINT('Origin',(-250.,-7.93749999999999,215.875));
#22142=CARTESIAN_POINT('',(-250.,-7.93749999999999,255.4625));
#22143=CARTESIAN_POINT('Origin',(-250.,-0.199999999999978,255.4625));
#22144=CARTESIAN_POINT('',(-250.,-0.199999999999978,263.2));
#22145=CARTESIAN_POINT('Origin',(-250.,0.,263.2));
#22146=CARTESIAN_POINT('Origin',(-340.039729762984,1.11022302462516E-13,
155.0625));
#22147=CARTESIAN_POINT('',(-349.039729762984,1.09920120343283E-13,155.0625));
#22148=CARTESIAN_POINT('Origin',(-340.039729762984,1.11022302462516E-13,
155.0625));
#22149=CARTESIAN_POINT('',(-349.039729762984,1.09920120343283E-13,163.));
#22150=CARTESIAN_POINT('',(-349.039729762984,1.09920120343283E-13,155.0625));
#22151=CARTESIAN_POINT('Origin',(-340.039729762984,0.,163.));
#22152=CARTESIAN_POINT('Origin',(-340.039729762984,1.11022302462516E-13,
155.0625));
#22153=CARTESIAN_POINT('',(-318.170320326478,-2.39351851851843,155.0625));
#22154=CARTESIAN_POINT('',(-340.039729762984,-21.9999999999999,155.0625));
#22155=CARTESIAN_POINT('Origin',(-340.039729762984,1.11022302462516E-13,
155.0625));
#22156=CARTESIAN_POINT('',(-340.039729762984,-22.,163.));
#22157=CARTESIAN_POINT('',(-340.039729762984,-21.9999999999999,155.0625));
#22158=CARTESIAN_POINT('',(-318.170320326478,-2.39351851851854,163.));
#22159=CARTESIAN_POINT('Origin',(-340.039729762984,0.,163.));
#22160=CARTESIAN_POINT('',(-318.170320326478,-2.39351851851843,155.0625));
#22161=CARTESIAN_POINT('Origin',(-313.2,-2.93749999999993,155.0625));
#22162=CARTESIAN_POINT('',(-313.2,-7.93749999999999,163.));
#22163=CARTESIAN_POINT('Origin',(-313.2,-2.93749999999998,163.));
#22164=CARTESIAN_POINT('',(-313.2,-7.93749999999988,155.0625));
#22165=CARTESIAN_POINT('',(-313.2,-7.93749999999988,155.0625));
#22166=CARTESIAN_POINT('Origin',(-313.2,-2.93749999999993,155.0625));
#22167=CARTESIAN_POINT('Origin',(-265.039729762984,-7.93749999999988,155.0625));
#22168=CARTESIAN_POINT('',(-265.039729762984,-7.93749999999999,163.));
#22169=CARTESIAN_POINT('',(-265.039729762984,-7.93749999999999,163.));
#22170=CARTESIAN_POINT('',(-265.039729762984,-7.93749999999988,155.0625));
#22171=CARTESIAN_POINT('',(-265.039729762984,-7.93749999999988,155.0625));
#22172=CARTESIAN_POINT('',(-265.039729762984,-7.93749999999988,155.0625));
#22173=CARTESIAN_POINT('Origin',(-260.039729762984,-12.9374999999999,155.0625));
#22174=CARTESIAN_POINT('',(-260.039729762984,-12.9375,163.));
#22175=CARTESIAN_POINT('',(-260.039729762984,-12.9375,163.));
#22176=CARTESIAN_POINT('',(-260.039729762984,-12.9374999999999,155.0625));
#22177=CARTESIAN_POINT('',(-260.039729762984,-12.9374999999999,155.0625));
#22178=CARTESIAN_POINT('',(-260.039729762984,-12.9374999999999,155.0625));
#22179=CARTESIAN_POINT('Origin',(-260.039729762984,-21.9999999999999,155.0625));
#22180=CARTESIAN_POINT('',(-260.039729762984,-22.,163.));
#22181=CARTESIAN_POINT('',(-260.039729762984,-22.,163.));
#22182=CARTESIAN_POINT('',(-260.039729762984,-21.9999999999999,155.0625));
#22183=CARTESIAN_POINT('',(-260.039729762984,-21.9999999999999,155.0625));
#22184=CARTESIAN_POINT('',(-260.039729762984,-21.9999999999999,155.0625));
#22185=CARTESIAN_POINT('Origin',(-340.039729762984,-21.9999999999999,155.0625));
#22186=CARTESIAN_POINT('',(-340.039729762984,-22.,163.));
#22187=CARTESIAN_POINT('',(-340.039729762984,-21.9999999999999,155.0625));
#22188=CARTESIAN_POINT('Origin',(-340.039729762984,1.11022302462516E-13,
155.0625));
#22189=CARTESIAN_POINT('Origin',(-340.039729762984,0.,163.));
#22190=CARTESIAN_POINT('Origin',(286.9375,-36.9375,178.55));
#22191=CARTESIAN_POINT('',(295.9375,-36.9375,178.55));
#22192=CARTESIAN_POINT('Origin',(286.9375,-36.9375,178.55));
#22193=CARTESIAN_POINT('',(295.9375,-36.9375,172.2));
#22194=CARTESIAN_POINT('',(295.9375,-36.9375,178.55));
#22195=CARTESIAN_POINT('Origin',(286.9375,-36.9375,172.2));
#22196=CARTESIAN_POINT('Origin',(286.9375,-36.9375,178.55));
#22197=CARTESIAN_POINT('',(265.875,-7.93749999999999,178.55));
#22198=CARTESIAN_POINT('',(257.9375,-15.874999999997,178.55));
#22199=CARTESIAN_POINT('',(257.9375,-15.874999999997,178.55));
#22200=CARTESIAN_POINT('',(257.9375,-55.9375,178.55));
#22201=CARTESIAN_POINT('',(257.9375,-55.9375,178.55));
#22202=CARTESIAN_POINT('',(286.9375,-55.9375,178.55));
#22203=CARTESIAN_POINT('',(286.9375,-55.9375,178.55));
#22204=CARTESIAN_POINT('',(305.9375,-36.9375,178.55));
#22205=CARTESIAN_POINT('Origin',(286.9375,-36.9375,178.55));
#22206=CARTESIAN_POINT('',(305.9375,-7.93749999999999,178.55));
#22207=CARTESIAN_POINT('',(305.9375,-7.93749999999999,178.55));
#22208=CARTESIAN_POINT('',(265.875,-7.93749999999999,178.55));
#22209=CARTESIAN_POINT('Origin',(286.9375,-36.9375,172.2));
#22210=CARTESIAN_POINT('',(265.875,-7.93749999999999,172.2));
#22211=CARTESIAN_POINT('',(257.9375,-15.874999999997,172.2));
#22212=CARTESIAN_POINT('',(257.9375,-15.874999999997,172.2));
#22213=CARTESIAN_POINT('',(305.9375,-7.93749999999999,172.2));
#22214=CARTESIAN_POINT('',(265.875,-7.93749999999999,172.2));
#22215=CARTESIAN_POINT('',(305.9375,-36.9375,172.2));
#22216=CARTESIAN_POINT('',(305.9375,-7.93749999999999,172.2));
#22217=CARTESIAN_POINT('',(286.9375,-55.9375,172.2));
#22218=CARTESIAN_POINT('Origin',(286.9375,-36.9375,172.2));
#22219=CARTESIAN_POINT('',(257.9375,-55.9375,172.2));
#22220=CARTESIAN_POINT('',(286.9375,-55.9375,172.2));
#22221=CARTESIAN_POINT('',(257.9375,-55.9375,172.2));
#22222=CARTESIAN_POINT('Origin',(257.9375,-15.874999999997,178.55));
#22223=CARTESIAN_POINT('',(257.9375,-15.874999999997,178.55));
#22224=CARTESIAN_POINT('',(265.875,-7.93749999999999,178.55));
#22225=CARTESIAN_POINT('Origin',(257.9375,-55.9375,178.55));
#22226=CARTESIAN_POINT('',(257.9375,-55.9375,178.55));
#22227=CARTESIAN_POINT('Origin',(286.9375,-55.9375,178.55));
#22228=CARTESIAN_POINT('',(286.9375,-55.9375,178.55));
#22229=CARTESIAN_POINT('Origin',(286.9375,-36.9375,178.55));
#22230=CARTESIAN_POINT('',(305.9375,-36.9375,178.55));
#22231=CARTESIAN_POINT('Origin',(305.9375,-7.93749999999999,178.55));
#22232=CARTESIAN_POINT('',(305.9375,-7.93749999999999,178.55));
#22233=CARTESIAN_POINT('Origin',(265.875,-7.93749999999999,178.55));
#22234=CARTESIAN_POINT('Origin',(-340.039729762984,0.,-155.0625));
#22235=CARTESIAN_POINT('',(-349.039729762984,1.10218211923262E-15,-155.0625));
#22236=CARTESIAN_POINT('Origin',(-340.039729762984,0.,-155.0625));
#22237=CARTESIAN_POINT('',(-349.039729762984,1.10218211923262E-15,-163.));
#22238=CARTESIAN_POINT('',(-349.039729762984,1.10218211923262E-15,-155.0625));
#22239=CARTESIAN_POINT('Origin',(-340.039729762984,0.,-163.));
#22240=CARTESIAN_POINT('Origin',(-340.039729762984,0.,-155.0625));
#22241=CARTESIAN_POINT('',(-318.170320326478,-2.39351851851849,-155.0625));
#22242=CARTESIAN_POINT('',(-340.039729762984,-22.,-155.0625));
#22243=CARTESIAN_POINT('Origin',(-340.039729762984,0.,-155.0625));
#22244=CARTESIAN_POINT('',(-318.170320326478,-2.39351851851849,-163.));
#22245=CARTESIAN_POINT('',(-318.170320326478,-2.39351851851849,-155.0625));
#22246=CARTESIAN_POINT('',(-340.039729762984,-22.,-163.));
#22247=CARTESIAN_POINT('Origin',(-340.039729762984,0.,-163.));
#22248=CARTESIAN_POINT('',(-340.039729762984,-22.,-155.0625));
#22249=CARTESIAN_POINT('Origin',(-313.2,-2.93749999999998,-155.0625));
#22250=CARTESIAN_POINT('',(-313.2,-7.93749999999999,-163.));
#22251=CARTESIAN_POINT('Origin',(-313.2,-2.93749999999998,-163.));
#22252=CARTESIAN_POINT('',(-313.2,-7.93749999999999,-155.0625));
#22253=CARTESIAN_POINT('Origin',(-313.2,-2.93749999999998,-155.0625));
#22254=CARTESIAN_POINT('',(-313.2,-7.93749999999999,-155.0625));
#22255=CARTESIAN_POINT('Origin',(-265.039729762984,-7.93749999999999,-155.0625));
#22256=CARTESIAN_POINT('',(-265.039729762984,-7.93749999999999,-163.));
#22257=CARTESIAN_POINT('',(-265.039729762984,-7.93749999999999,-163.));
#22258=CARTESIAN_POINT('',(-265.039729762984,-7.93749999999999,-155.0625));
#22259=CARTESIAN_POINT('',(-265.039729762984,-7.93749999999999,-155.0625));
#22260=CARTESIAN_POINT('',(-265.039729762984,-7.93749999999999,-155.0625));
#22261=CARTESIAN_POINT('Origin',(-260.039729762984,-12.9374999999999,-155.0625));
#22262=CARTESIAN_POINT('',(-260.039729762984,-12.9374999999999,-163.));
#22263=CARTESIAN_POINT('',(-260.039729762984,-12.9374999999999,-163.));
#22264=CARTESIAN_POINT('',(-260.039729762984,-12.9374999999999,-155.0625));
#22265=CARTESIAN_POINT('',(-260.039729762984,-12.9374999999999,-155.0625));
#22266=CARTESIAN_POINT('',(-260.039729762984,-12.9374999999999,-155.0625));
#22267=CARTESIAN_POINT('Origin',(-260.039729762984,-22.,-155.0625));
#22268=CARTESIAN_POINT('',(-260.039729762984,-22.,-163.));
#22269=CARTESIAN_POINT('',(-260.039729762984,-22.,-163.));
#22270=CARTESIAN_POINT('',(-260.039729762984,-22.,-155.0625));
#22271=CARTESIAN_POINT('',(-260.039729762984,-22.,-155.0625));
#22272=CARTESIAN_POINT('',(-260.039729762984,-22.,-155.0625));
#22273=CARTESIAN_POINT('Origin',(-340.039729762984,-22.,-155.0625));
#22274=CARTESIAN_POINT('',(-340.039729762984,-22.,-163.));
#22275=CARTESIAN_POINT('',(-340.039729762984,-22.,-155.0625));
#22276=CARTESIAN_POINT('Origin',(-340.039729762984,0.,-155.0625));
#22277=CARTESIAN_POINT('Origin',(-340.039729762984,0.,-163.));
#22278=CARTESIAN_POINT('Origin',(286.9375,-36.9375,-178.55));
#22279=CARTESIAN_POINT('',(295.9375,-36.9375,-178.55));
#22280=CARTESIAN_POINT('Origin',(286.9375,-36.9375,-178.55));
#22281=CARTESIAN_POINT('',(295.9375,-36.9375,-172.2));
#22282=CARTESIAN_POINT('',(295.9375,-36.9375,-178.55));
#22283=CARTESIAN_POINT('Origin',(286.9375,-36.9375,-172.2));
#22284=CARTESIAN_POINT('Origin',(286.9375,-36.9375,-178.55));
#22285=CARTESIAN_POINT('',(265.875,-7.93749999999999,-178.55));
#22286=CARTESIAN_POINT('',(257.9375,-15.874999999997,-178.55));
#22287=CARTESIAN_POINT('',(257.9375,-15.874999999997,-178.55));
#22288=CARTESIAN_POINT('',(305.9375,-7.93749999999999,-178.55));
#22289=CARTESIAN_POINT('',(265.875,-7.93749999999999,-178.55));
#22290=CARTESIAN_POINT('',(305.9375,-36.9375,-178.55));
#22291=CARTESIAN_POINT('',(305.9375,-7.93749999999999,-178.55));
#22292=CARTESIAN_POINT('',(286.9375,-55.9375,-178.55));
#22293=CARTESIAN_POINT('Origin',(286.9375,-36.9375,-178.55));
#22294=CARTESIAN_POINT('',(257.9375,-55.9375,-178.55));
#22295=CARTESIAN_POINT('',(286.9375,-55.9375,-178.55));
#22296=CARTESIAN_POINT('',(257.9375,-55.9375,-178.55));
#22297=CARTESIAN_POINT('Origin',(286.9375,-36.9375,-172.2));
#22298=CARTESIAN_POINT('',(265.875,-7.93749999999999,-172.2));
#22299=CARTESIAN_POINT('',(257.9375,-15.874999999997,-172.2));
#22300=CARTESIAN_POINT('',(257.9375,-15.874999999997,-172.2));
#22301=CARTESIAN_POINT('',(257.9375,-55.9375,-172.2));
#22302=CARTESIAN_POINT('',(257.9375,-55.9375,-172.2));
#22303=CARTESIAN_POINT('',(286.9375,-55.9375,-172.2));
#22304=CARTESIAN_POINT('',(286.9375,-55.9375,-172.2));
#22305=CARTESIAN_POINT('',(305.9375,-36.9375,-172.2));
#22306=CARTESIAN_POINT('Origin',(286.9375,-36.9375,-172.2));
#22307=CARTESIAN_POINT('',(305.9375,-7.93749999999999,-172.2));
#22308=CARTESIAN_POINT('',(305.9375,-7.93749999999999,-172.2));
#22309=CARTESIAN_POINT('',(265.875,-7.93749999999999,-172.2));
#22310=CARTESIAN_POINT('Origin',(257.9375,-15.874999999997,-178.55));
#22311=CARTESIAN_POINT('',(265.875,-7.93749999999999,-178.55));
#22312=CARTESIAN_POINT('',(257.9375,-15.874999999997,-178.55));
#22313=CARTESIAN_POINT('Origin',(257.9375,-55.9375,-178.55));
#22314=CARTESIAN_POINT('',(257.9375,-55.9375,-178.55));
#22315=CARTESIAN_POINT('Origin',(286.9375,-55.9375,-178.55));
#22316=CARTESIAN_POINT('',(286.9375,-55.9375,-178.55));
#22317=CARTESIAN_POINT('Origin',(286.9375,-36.9375,-178.55));
#22318=CARTESIAN_POINT('',(305.9375,-36.9375,-178.55));
#22319=CARTESIAN_POINT('Origin',(305.9375,-7.93749999999999,-178.55));
#22320=CARTESIAN_POINT('',(305.9375,-7.93749999999999,-178.55));
#22321=CARTESIAN_POINT('Origin',(265.875,-7.93749999999999,-178.55));
#22322=CARTESIAN_POINT('Origin',(284.2,-10.000000000002,-163.2));
#22323=CARTESIAN_POINT('',(284.2,-7.93749999999716,-154.2));
#22324=CARTESIAN_POINT('',(284.2,-7.93749999999716,-172.2));
#22325=CARTESIAN_POINT('Origin',(284.2,-7.9374999999971,-163.2));
#22326=CARTESIAN_POINT('',(284.2,-1.99840144432528E-12,-172.2));
#22327=CARTESIAN_POINT('',(284.2,-10.000000000002,-172.2));
#22328=CARTESIAN_POINT('',(284.2,-1.99840144432528E-12,-154.2));
#22329=CARTESIAN_POINT('Origin',(284.2,-1.99840144432528E-12,-163.2));
#22330=CARTESIAN_POINT('',(284.2,-10.000000000002,-154.2));
#22331=CARTESIAN_POINT('Origin',(284.2,-10.000000000002,163.2));
#22332=CARTESIAN_POINT('',(284.2,-7.93749999999716,172.2));
#22333=CARTESIAN_POINT('',(284.2,-7.93749999999704,154.2));
#22334=CARTESIAN_POINT('Origin',(284.2,-7.9374999999971,163.2));
#22335=CARTESIAN_POINT('',(284.2,-1.88737914186277E-12,154.2));
#22336=CARTESIAN_POINT('',(284.2,-10.0000000000019,154.2));
#22337=CARTESIAN_POINT('',(284.2,-1.99840144432528E-12,172.2));
#22338=CARTESIAN_POINT('Origin',(284.2,-1.99840144432528E-12,163.2));
#22339=CARTESIAN_POINT('',(284.2,-10.000000000002,172.2));
#22340=CARTESIAN_POINT('Origin',(305.4625,-0.199999999997258,200.));
#22341=CARTESIAN_POINT('',(313.2,-0.199999999997258,-154.2));
#22342=CARTESIAN_POINT('',(305.4625,-7.93749999999721,-154.2));
#22343=CARTESIAN_POINT('Origin',(305.4625,-0.199999999997202,-154.2));
#22344=CARTESIAN_POINT('',(313.2,-0.199999999997202,154.2));
#22345=CARTESIAN_POINT('',(313.2,-0.199999999997258,200.));
#22346=CARTESIAN_POINT('',(305.4625,-7.93749999999716,154.2));
#22347=CARTESIAN_POINT('Origin',(305.4625,-0.199999999997147,154.2));
#22348=CARTESIAN_POINT('',(305.4625,-7.93749999999721,200.));
#22349=CARTESIAN_POINT('Origin',(305.4625,-0.199999999997258,200.));
#22350=CARTESIAN_POINT('',(313.2,-0.199999999997313,172.2));
#22351=CARTESIAN_POINT('',(305.4625,-7.93749999999727,172.2));
#22352=CARTESIAN_POINT('Origin',(305.4625,-0.199999999997258,172.2));
#22353=CARTESIAN_POINT('',(313.2,-0.199999999997258,263.2));
#22354=CARTESIAN_POINT('',(313.2,-0.199999999997258,200.));
#22355=CARTESIAN_POINT('',(305.4625,-7.93749999999721,255.4625));
#22356=CARTESIAN_POINT('Origin',(305.462500000002,-0.199999999999014,255.462500000001));
#22357=CARTESIAN_POINT('',(305.4625,-7.93749999999721,200.));
#22358=CARTESIAN_POINT('Origin',(313.2,2.72004641033163E-12,200.));
#22359=CARTESIAN_POINT('',(313.2,-2.22044604925031E-12,-154.2));
#22360=CARTESIAN_POINT('',(313.2,2.72004641033163E-12,-154.2));
#22361=CARTESIAN_POINT('',(313.2,-2.1094237467878E-12,154.2));
#22362=CARTESIAN_POINT('',(313.2,2.72004641033163E-12,200.));
#22363=CARTESIAN_POINT('',(313.2,2.77555756156289E-12,154.2));
#22364=CARTESIAN_POINT('Origin',(313.2,2.72004641033163E-12,200.));
#22365=CARTESIAN_POINT('',(313.2,-2.22044604925031E-12,172.2));
#22366=CARTESIAN_POINT('',(313.2,2.72004641033163E-12,172.2));
#22367=CARTESIAN_POINT('',(313.2,2.72004641033163E-12,263.2));
#22368=CARTESIAN_POINT('',(313.2,2.72004641033163E-12,200.));
#22369=CARTESIAN_POINT('',(313.2,2.27595720048157E-12,263.2));
#22370=CARTESIAN_POINT('Origin',(250.,0.,-200.));
#22371=CARTESIAN_POINT('',(313.2,-0.199999999997202,-263.2));
#22372=CARTESIAN_POINT('',(313.2,2.77555756156289E-12,-263.2));
#22373=CARTESIAN_POINT('',(313.2,6.0507154842071E-12,-263.2));
#22374=CARTESIAN_POINT('',(305.4625,-7.93749999999716,-255.4625));
#22375=CARTESIAN_POINT('Origin',(305.462499999999,-0.199999999996119,-255.462499999999));
#22376=CARTESIAN_POINT('',(265.875,-7.93749999999699,-215.875));
#22377=CARTESIAN_POINT('',(57.9375,-7.93749999999554,-7.93749999999999));
#22378=CARTESIAN_POINT('',(257.9375,-15.8749999999969,-207.9375));
#22379=CARTESIAN_POINT('Origin',(265.875000000002,-15.8749999999988,-215.875000000002));
#22380=CARTESIAN_POINT('',(257.9375,-55.4624999999969,-207.9375));
#22381=CARTESIAN_POINT('',(257.9375,-55.4624999999969,-207.9375));
#22382=CARTESIAN_POINT('',(250.2,-63.1999999999969,-200.2));
#22383=CARTESIAN_POINT('Origin',(250.200000000003,-55.4625000000002,-200.200000000003));
#22384=CARTESIAN_POINT('',(250.,-63.1999999999969,-200.));
#22385=CARTESIAN_POINT('',(49.9999999999996,-63.1999999999969,0.));
#22386=CARTESIAN_POINT('',(250.,3.1641356201817E-12,-200.));
#22387=CARTESIAN_POINT('',(250.,3.10862446895044E-12,-200.));
#22388=CARTESIAN_POINT('',(81.6,4.32986979603811E-12,-31.6));
#22389=CARTESIAN_POINT('Origin',(250.,0.,200.));
#22390=CARTESIAN_POINT('',(250.,3.1641356201817E-12,200.));
#22391=CARTESIAN_POINT('',(281.6,2.94209101525666E-12,231.6));
#22392=CARTESIAN_POINT('',(250.,-63.1999999999969,200.));
#22393=CARTESIAN_POINT('',(250.,3.1641356201817E-12,200.));
#22394=CARTESIAN_POINT('',(250.2,-63.1999999999969,200.199999999999));
#22395=CARTESIAN_POINT('',(250.,-63.1999999999969,200.));
#22396=CARTESIAN_POINT('',(257.9375,-55.4624999999969,207.937499999999));
#22397=CARTESIAN_POINT('Origin',(250.200000000002,-55.4624999999997,200.200000000002));
#22398=CARTESIAN_POINT('',(257.9375,-15.8749999999969,207.9375));
#22399=CARTESIAN_POINT('',(257.9375,-55.462499999997,207.937499999999));
#22400=CARTESIAN_POINT('',(265.875,-7.93749999999693,215.875));
#22401=CARTESIAN_POINT('Origin',(265.875,-15.8749999999973,215.875));
#22402=CARTESIAN_POINT('',(257.9375,-7.93749999999688,207.9375));
#22403=CARTESIAN_POINT('Origin',(313.2,2.72004641033163E-12,200.));
#22404=CARTESIAN_POINT('',(342.2,-2.38697950294409E-12,-154.2));
#22405=CARTESIAN_POINT('',(313.2,-2.22044604925031E-12,-172.2));
#22406=CARTESIAN_POINT('',(342.2,-2.38697950294409E-12,-172.2));
#22407=CARTESIAN_POINT('',(313.2,2.72004641033163E-12,200.));
#22408=CARTESIAN_POINT('',(250.,3.1641356201817E-12,200.));
#22409=CARTESIAN_POINT('',(342.2,-2.44249065417534E-12,172.2));
#22410=CARTESIAN_POINT('',(342.2,-2.33146835171283E-12,154.2));
#22411=CARTESIAN_POINT('Origin',(250.,3.1641356201817E-12,200.));
#22412=CARTESIAN_POINT('',(250.,-63.1999999999969,200.));
#22413=CARTESIAN_POINT('Origin',(250.,-63.1999999999969,200.));
#22414=CARTESIAN_POINT('',(250.2,-63.1999999999969,200.));
#22415=CARTESIAN_POINT('Origin',(250.2,-55.4624999999969,200.));
#22416=CARTESIAN_POINT('',(257.9375,-55.4624999999969,200.));
#22417=CARTESIAN_POINT('Origin',(257.9375,-55.4624999999969,200.));
#22418=CARTESIAN_POINT('',(257.9375,-15.8749999999969,200.));
#22419=CARTESIAN_POINT('Origin',(265.875,-15.874999999997,200.));
#22420=CARTESIAN_POINT('',(265.875,-7.93749999999693,200.));
#22421=CARTESIAN_POINT('Origin',(265.875,-7.93749999999699,200.));
#22422=CARTESIAN_POINT('',(265.875,-7.93749999999693,-154.2));
#22423=CARTESIAN_POINT('',(265.875,-7.93749999999688,154.2));
#22424=CARTESIAN_POINT('',(265.875,-7.93749999999699,172.2));
#22425=CARTESIAN_POINT('',(305.4625,-7.93749999999727,-172.2));
#22426=CARTESIAN_POINT('',(305.4625,-7.93749999999721,200.));
#22427=CARTESIAN_POINT('',(265.875,-7.93749999999693,-172.2));
#22428=CARTESIAN_POINT('Origin',(305.4625,-0.199999999997258,200.));
#22429=CARTESIAN_POINT('',(313.2,-0.199999999997258,-172.2));
#22430=CARTESIAN_POINT('Origin',(305.4625,-0.199999999997258,-172.2));
#22431=CARTESIAN_POINT('',(313.2,-0.199999999997258,200.));
#22432=CARTESIAN_POINT('Origin',(313.2,2.72004641033163E-12,200.));
#22433=CARTESIAN_POINT('',(313.2,2.72004641033163E-12,-172.2));
#22434=CARTESIAN_POINT('Origin',(342.2,-10.0000000000024,172.2));
#22435=CARTESIAN_POINT('Origin',(342.2,-10.0000000000023,154.2));
#22436=CARTESIAN_POINT('Origin',(342.2,-10.0000000000024,-154.2));
#22437=CARTESIAN_POINT('Origin',(342.2,-10.0000000000024,-172.2));
#22438=CARTESIAN_POINT('Origin',(286.9375,-36.9374999999999,147.85));
#22439=CARTESIAN_POINT('',(295.9375,-36.9374999999999,147.85));
#22440=CARTESIAN_POINT('Origin',(286.9375,-36.9374999999999,147.85));
#22441=CARTESIAN_POINT('',(295.9375,-36.9374999999999,154.2));
#22442=CARTESIAN_POINT('',(295.9375,-36.9374999999999,147.85));
#22443=CARTESIAN_POINT('Origin',(286.9375,-36.9374999999999,154.2));
#22444=CARTESIAN_POINT('Origin',(286.9375,-36.9374999999999,147.85));
#22445=CARTESIAN_POINT('',(265.875,-7.93749999999988,147.85));
#22446=CARTESIAN_POINT('',(257.9375,-15.8749999999969,147.85));
#22447=CARTESIAN_POINT('',(257.9375,-15.8749999999969,147.85));
#22448=CARTESIAN_POINT('',(305.9375,-7.93749999999988,147.85));
#22449=CARTESIAN_POINT('',(265.875,-7.93749999999988,147.85));
#22450=CARTESIAN_POINT('',(305.9375,-36.9374999999999,147.85));
#22451=CARTESIAN_POINT('',(305.9375,-7.93749999999988,147.85));
#22452=CARTESIAN_POINT('',(286.9375,-55.9374999999999,147.85));
#22453=CARTESIAN_POINT('Origin',(286.9375,-36.9374999999999,147.85));
#22454=CARTESIAN_POINT('',(257.9375,-55.9374999999999,147.85));
#22455=CARTESIAN_POINT('',(286.9375,-55.9374999999999,147.85));
#22456=CARTESIAN_POINT('',(257.9375,-55.9374999999999,147.85));
#22457=CARTESIAN_POINT('Origin',(286.9375,-36.9374999999999,154.2));
#22458=CARTESIAN_POINT('',(265.875,-7.93749999999988,154.2));
#22459=CARTESIAN_POINT('',(257.9375,-15.8749999999969,154.2));
#22460=CARTESIAN_POINT('',(257.9375,-15.8749999999969,154.2));
#22461=CARTESIAN_POINT('',(257.9375,-55.9374999999999,154.2));
#22462=CARTESIAN_POINT('',(257.9375,-55.9374999999999,154.2));
#22463=CARTESIAN_POINT('',(286.9375,-55.9374999999999,154.2));
#22464=CARTESIAN_POINT('',(286.9375,-55.9374999999999,154.2));
#22465=CARTESIAN_POINT('',(305.9375,-36.9374999999999,154.2));
#22466=CARTESIAN_POINT('Origin',(286.9375,-36.9374999999999,154.2));
#22467=CARTESIAN_POINT('',(305.9375,-7.93749999999988,154.2));
#22468=CARTESIAN_POINT('',(305.9375,-7.93749999999988,154.2));
#22469=CARTESIAN_POINT('',(265.875,-7.93749999999988,154.2));
#22470=CARTESIAN_POINT('Origin',(257.9375,-15.8749999999969,147.85));
#22471=CARTESIAN_POINT('',(265.875,-7.93749999999988,147.85));
#22472=CARTESIAN_POINT('',(257.9375,-15.8749999999969,147.85));
#22473=CARTESIAN_POINT('Origin',(257.9375,-55.9374999999999,147.85));
#22474=CARTESIAN_POINT('',(257.9375,-55.9374999999999,147.85));
#22475=CARTESIAN_POINT('Origin',(286.9375,-55.9374999999999,147.85));
#22476=CARTESIAN_POINT('',(286.9375,-55.9374999999999,147.85));
#22477=CARTESIAN_POINT('Origin',(286.9375,-36.9374999999999,147.85));
#22478=CARTESIAN_POINT('',(305.9375,-36.9374999999999,147.85));
#22479=CARTESIAN_POINT('Origin',(305.9375,-7.93749999999988,147.85));
#22480=CARTESIAN_POINT('',(305.9375,-7.93749999999988,147.85));
#22481=CARTESIAN_POINT('Origin',(265.875,-7.93749999999988,147.85));
#22482=CARTESIAN_POINT('Origin',(286.9375,-36.9375,-147.85));
#22483=CARTESIAN_POINT('',(295.9375,-36.9375,-147.85));
#22484=CARTESIAN_POINT('Origin',(286.9375,-36.9375,-147.85));
#22485=CARTESIAN_POINT('',(295.9375,-36.9375,-154.2));
#22486=CARTESIAN_POINT('',(295.9375,-36.9375,-147.85));
#22487=CARTESIAN_POINT('Origin',(286.9375,-36.9375,-154.2));
#22488=CARTESIAN_POINT('Origin',(286.9375,-36.9375,-147.85));
#22489=CARTESIAN_POINT('',(265.875,-7.93749999999999,-147.85));
#22490=CARTESIAN_POINT('',(257.9375,-15.8749999999969,-147.85));
#22491=CARTESIAN_POINT('',(257.9375,-15.8749999999969,-147.85));
#22492=CARTESIAN_POINT('',(257.9375,-55.9375,-147.85));
#22493=CARTESIAN_POINT('',(257.9375,-55.9375,-147.85));
#22494=CARTESIAN_POINT('',(286.9375,-55.9375,-147.85));
#22495=CARTESIAN_POINT('',(286.9375,-55.9375,-147.85));
#22496=CARTESIAN_POINT('',(305.9375,-36.9375,-147.85));
#22497=CARTESIAN_POINT('Origin',(286.9375,-36.9375,-147.85));
#22498=CARTESIAN_POINT('',(305.9375,-7.93749999999999,-147.85));
#22499=CARTESIAN_POINT('',(305.9375,-7.93749999999999,-147.85));
#22500=CARTESIAN_POINT('',(265.875,-7.93749999999999,-147.85));
#22501=CARTESIAN_POINT('Origin',(286.9375,-36.9375,-154.2));
#22502=CARTESIAN_POINT('',(265.875,-7.93749999999999,-154.2));
#22503=CARTESIAN_POINT('',(257.9375,-15.874999999997,-154.2));
#22504=CARTESIAN_POINT('',(257.9375,-15.874999999997,-154.2));
#22505=CARTESIAN_POINT('',(305.9375,-7.93749999999999,-154.2));
#22506=CARTESIAN_POINT('',(265.875,-7.93749999999999,-154.2));
#22507=CARTESIAN_POINT('',(305.9375,-36.9375,-154.2));
#22508=CARTESIAN_POINT('',(305.9375,-7.93749999999999,-154.2));
#22509=CARTESIAN_POINT('',(286.9375,-55.9375,-154.2));
#22510=CARTESIAN_POINT('Origin',(286.9375,-36.9375,-154.2));
#22511=CARTESIAN_POINT('',(257.9375,-55.9375,-154.2));
#22512=CARTESIAN_POINT('',(286.9375,-55.9375,-154.2));
#22513=CARTESIAN_POINT('',(257.9375,-55.9375,-154.2));
#22514=CARTESIAN_POINT('Origin',(257.9375,-15.8749999999969,-147.85));
#22515=CARTESIAN_POINT('',(257.9375,-15.8749999999969,-147.85));
#22516=CARTESIAN_POINT('',(265.875,-7.93749999999999,-147.85));
#22517=CARTESIAN_POINT('Origin',(257.9375,-55.9375,-147.85));
#22518=CARTESIAN_POINT('',(257.9375,-55.9375,-147.85));
#22519=CARTESIAN_POINT('Origin',(286.9375,-55.9375,-147.85));
#22520=CARTESIAN_POINT('',(286.9375,-55.9375,-147.85));
#22521=CARTESIAN_POINT('Origin',(286.9375,-36.9375,-147.85));
#22522=CARTESIAN_POINT('',(305.9375,-36.9375,-147.85));
#22523=CARTESIAN_POINT('Origin',(305.9375,-7.93749999999999,-147.85));
#22524=CARTESIAN_POINT('',(305.9375,-7.93749999999999,-147.85));
#22525=CARTESIAN_POINT('Origin',(265.875,-7.93749999999999,-147.85));
#32874=UNCERTAINTY_MEASURE_WITH_UNIT(LENGTH_MEASURE(0.01),#32904,
'DISTANCE_ACCURACY_VALUE',
'Maximum model space distance between geometric entities at asserted c
onnectivities');
#32886=UNCERTAINTY_MEASURE_WITH_UNIT(LENGTH_MEASURE(0.01),#32904,
'DISTANCE_ACCURACY_VALUE',
'Maximum model space distance between geometric entities at asserted c
onnectivities');
#32891=(
GEOMETRIC_REPRESENTATION_CONTEXT(3)
GLOBAL_UNCERTAINTY_ASSIGNED_CONTEXT((#32874))
GLOBAL_UNIT_ASSIGNED_CONTEXT((#32904,#32906,#32907))
REPRESENTATION_CONTEXT('','3D')
);
#32903=(
GEOMETRIC_REPRESENTATION_CONTEXT(3)
GLOBAL_UNCERTAINTY_ASSIGNED_CONTEXT((#32886))
GLOBAL_UNIT_ASSIGNED_CONTEXT((#32904,#32906,#32907))
REPRESENTATION_CONTEXT('','3D')
);
#32904=(
LENGTH_UNIT()
NAMED_UNIT(*)
SI_UNIT(.MILLI.,.METRE.)
);
#32906=(
NAMED_UNIT(*)
PLANE_ANGLE_UNIT()
SI_UNIT($,.RADIAN.)
);
#32907=(
NAMED_UNIT(*)
SI_UNIT($,.STERADIAN.)
SOLID_ANGLE_UNIT()
);
#32912=SHAPE_DEFINITION_REPRESENTATION(#32928,#33016);
#32928=PRODUCT_DEFINITION_SHAPE('',$,#33033);
#33016=SHAPE_REPRESENTATION('',(#16041),#32891);
#33028=PRODUCT_DEFINITION_CONTEXT('part definition',#33078,'design');
#33033=PRODUCT_DEFINITION('Access Door Frame','Access Door Frame',#33049,
#33028);
#33049=PRODUCT_DEFINITION_FORMATION('',$,#33084);
#33078=APPLICATION_CONTEXT(
'Core Data for Automotive Mechanical Design Process');
#33079=PRODUCT_CONTEXT('part definition',#33078,'mechanical');
#33084=PRODUCT('Access Door Frame','Access Door Frame',$,(#33079));
#33098=PRESENTATION_STYLE_ASSIGNMENT((#33104));
#33104=SURFACE_STYLE_USAGE(.BOTH.,#33110);
#33110=SURFACE_SIDE_STYLE('',(#33116));
#33116=SURFACE_STYLE_FILL_AREA(#33122);
#33122=FILL_AREA_STYLE('Opaque(227,224,212)',(#33128));
#33128=FILL_AREA_STYLE_COLOUR('Opaque(227,224,212)',#33134);
#33134=COLOUR_RGB('Opaque(227,224,212)',0.890196078431372,0.87843137254902,
0.831372549019608);
ENDSEC;
END-ISO-10303-21;
